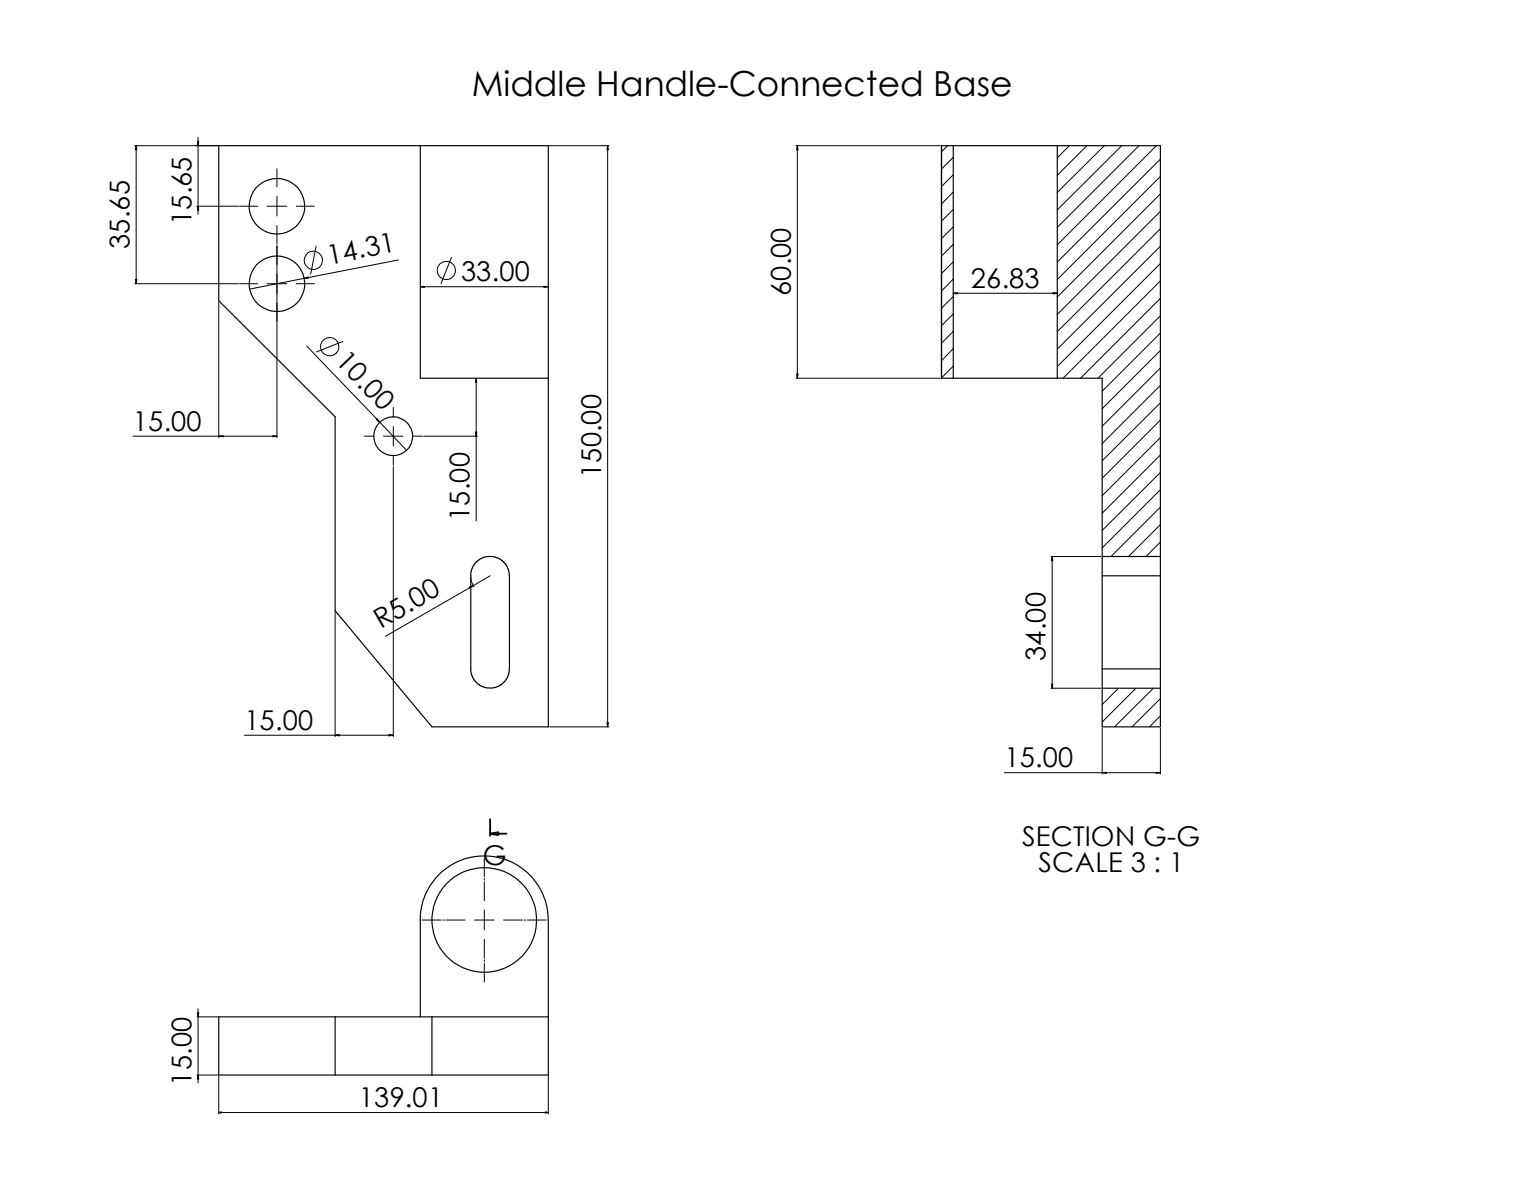
ISO-10303-21;
HEADER;
FILE_DESCRIPTION (('STEP AP214'),
    '1' );
FILE_NAME ('Middle Handle-Connected Base.step',
    '2026-10-26T22:46:44',
    ( '' ),
    ( '' ),
    'SwSTEP 2.0',
    'SolidWorks 2025',
    '' );
FILE_SCHEMA (( 'AUTOMOTIVE_DESIGN' ));
ENDSEC;

DATA;
#80=VECTOR ( 'NONE', #13900, 1000.000000000000227 ) ;
#95=DIRECTION ( 'NONE',  ( -0.5000000000000042188, 0.8660254037844362651, -2.168404344971015524E-16 ) ) ;
#104=EDGE_CURVE ( 'NONE', #402, #10896, #9651, .T. ) ;
#124=CYLINDRICAL_SURFACE ( 'NONE', #4697, 7.155882939242642848 ) ;
#181=EDGE_LOOP ( 'NONE', ( #14178, #14869, #3890, #5041 ) ) ;
#191=ORIENTED_EDGE ( 'NONE', *, *, #11432, .T. ) ;
#206=VERTEX_POINT ( 'NONE', #13865 ) ;
#216=ORIENTED_EDGE ( 'NONE', *, *, #15468, .T. ) ;
#231=DIRECTION ( 'NONE',  ( 0.8660254037844360431, 0.5000000000000044409, -5.976026924694052093E-17 ) ) ;
#281=ORIENTED_EDGE ( 'NONE', *, *, #10002, .F. ) ;
#314=DIRECTION ( 'NONE',  ( 0.5000000000000051070, -0.8660254037844358210, 0.000000000000000000 ) ) ;
#366=ORIENTED_EDGE ( 'NONE', *, *, #15468, .F. ) ;
#398=AXIS2_PLACEMENT_3D ( 'NONE', #14212, #20751, #11112 ) ;
#399=CARTESIAN_POINT ( 'NONE',  ( 77.00490953756757051, 160.5799536996104564, 56.00000000000000711 ) ) ;
#402=VERTEX_POINT ( 'NONE', #14604 ) ;
#403=LINE ( 'NONE', #2101, #20013 ) ;
#458=CARTESIAN_POINT ( 'NONE',  ( 63.15554463217812042, 234.5677573683057062, -19.00000000000000355 ) ) ;
#558=PLANE ( 'NONE',  #15135 ) ;
#564=DIRECTION ( 'NONE',  ( -0.8660254037844359321, -0.5000000000000045519, 5.976026924694053325E-17 ) ) ;
#607=ORIENTED_EDGE ( 'NONE', *, *, #16305, .F. ) ;
#611=CARTESIAN_POINT ( 'NONE',  ( 44.00490953756722945, 217.7376303493834087, -14.00000000000002842 ) ) ;
#722=DIRECTION ( 'NONE',  ( 0.5000000000000042188, -0.8660254037844362651, 1.445602896647343847E-16 ) ) ;
#732=DIRECTION ( 'NONE',  ( 0.000000000000000000, -1.000000000000000000, 2.176694594656153859E-16 ) ) ;
#771=CARTESIAN_POINT ( 'NONE',  ( 22.00490953756706958, 255.8427481158984165, 1.000000000000018208 ) ) ;
#848=ADVANCED_FACE ( 'NONE', ( #20058 ), #558, .F. ) ;
#853=DIRECTION ( 'NONE',  ( -0.5000000000000045519, 0.8660254037844361541, 0.000000000000000000 ) ) ;
#897=ORIENTED_EDGE ( 'NONE', *, *, #5211, .T. ) ;
#898=UNCERTAINTY_MEASURE_WITH_UNIT (LENGTH_MEASURE( 1.000000000000000082E-05 ), #14114, 'distance_accuracy_value', 'NONE');
#903=ORIENTED_EDGE ( 'NONE', *, *, #20153, .T. ) ;
#929=DIRECTION ( 'NONE',  ( -0.8660254037844363761, -0.5000000000000041078, -0.000000000000000000 ) ) ;
#936=CIRCLE ( 'NONE', #18890, 13.50000000000000711 ) ;
#966=EDGE_LOOP ( 'NONE', ( #19200, #16679, #7135, #19433, #20564 ) ) ;
#970=VECTOR ( 'NONE', #19207, 1000.000000000000227 ) ;
#992=EDGE_CURVE ( 'NONE', #997, #5249, #4157, .T. ) ;
#997=VERTEX_POINT ( 'NONE', #771 ) ;
#1026=CARTESIAN_POINT ( 'NONE',  ( 74.05523633728022048, 112.6889375482328717, -12.50000000000000000 ) ) ;
#1127=CIRCLE ( 'NONE', #4512, 7.155882939242646401 ) ;
#1161=ORIENTED_EDGE ( 'NONE', *, *, #19027, .T. ) ;
#1196=EDGE_CURVE ( 'NONE', #9961, #1291, #4537, .T. ) ;
#1200=CYLINDRICAL_SURFACE ( 'NONE', #16859, 5.000000000000033751 ) ;
#1201=VERTEX_POINT ( 'NONE', #3093 ) ;
#1233=FACE_BOUND ( 'NONE', #5689, .T. ) ;
#1259=CARTESIAN_POINT ( 'NONE',  ( 37.00490953756720813, 229.8619860023653132, 26.00000000000001776 ) ) ;
#1274=DIRECTION ( 'NONE',  ( 0.000000000000000000, 0.000000000000000000, 1.000000000000000000 ) ) ;
#1291=VERTEX_POINT ( 'NONE', #4976 ) ;
#1320=EDGE_CURVE ( 'NONE', #8085, #4151, #16435, .T. ) ;
#1358=CARTESIAN_POINT ( 'NONE',  ( 76.19073749086850000, 131.9901410505959518, 41.00000000000001421 ) ) ;
#1365=CARTESIAN_POINT ( 'NONE',  ( 57.00490953756744972, 195.2209698509878990, 11.00000000000001066 ) ) ;
#1416=FACE_BOUND ( 'NONE', #7340, .T. ) ;
#1436=FACE_OUTER_BOUND ( 'NONE', #3782, .T. ) ;
#1538=DIRECTION ( 'NONE',  ( -0.000000000000000000, -0.000000000000000000, 1.000000000000000000 ) ) ;
#1542=CARTESIAN_POINT ( 'NONE',  ( 54.01452848080093361, 170.4004617752990498, 4.000000000000000000 ) ) ;
#1577=ORIENTED_EDGE ( 'NONE', *, *, #12902, .F. ) ;
#1610=CARTESIAN_POINT ( 'NONE',  ( 32.36389338619004263, 157.9004617752989930, -12.50000000000000000 ) ) ;
#1616=EDGE_CURVE ( 'NONE', #1291, #10896, #11018, .T. ) ;
#1617=ORIENTED_EDGE ( 'NONE', *, *, #16795, .T. ) ;
#1641=DIRECTION ( 'NONE',  ( 0.5000000000000044409, -0.8660254037844360431, -0.000000000000000000 ) ) ;
#1651=CARTESIAN_POINT ( 'NONE',  ( 57.02433875312727452, 129.1873174624876413, 41.00000000000001421 ) ) ;
#1654=CARTESIAN_POINT ( 'NONE',  ( 44.05523633727993627, 164.6504617752990498, -12.50000000000000000 ) ) ;
#1656=VERTEX_POINT ( 'NONE', #3646 ) ;
#1676=DIRECTION ( 'NONE',  ( 0.5000000000000051070, -0.8660254037844358210, 0.000000000000000000 ) ) ;
#1741=EDGE_CURVE ( 'NONE', #17881, #8280, #5547, .T. ) ;
#1819=DIRECTION ( 'NONE',  ( 0.8660254037844360431, 0.5000000000000044409, -5.976026924694053325E-17 ) ) ;
#1881=EDGE_CURVE ( 'NONE', #997, #17881, #20600, .T. ) ;
#1891=ORIENTED_EDGE ( 'NONE', *, *, #4582, .T. ) ;
#1918=DIRECTION ( 'NONE',  ( 0.3535533905932770060, -0.6123724356957921389, 0.7071067811865480168 ) ) ;
#1924=VECTOR ( 'NONE', #8304, 1000.000000000000227 ) ;
#1928=CARTESIAN_POINT ( 'NONE',  ( 89.18111854763502322, 139.4901410505960087, 41.00000000000001421 ) ) ;
#1943=( NAMED_UNIT ( * ) SI_UNIT ( $, .STERADIAN. ) SOLID_ANGLE_UNIT ( ) );
#1948=EDGE_CURVE ( 'NONE', #10896, #402, #5560, .T. ) ;
#2017=DIRECTION ( 'NONE',  ( -0.8660254037844359321, -0.5000000000000045519, 5.976026924694053325E-17 ) ) ;
#2094=VECTOR ( 'NONE', #16006, 1000.000000000000227 ) ;
#2101=CARTESIAN_POINT ( 'NONE',  ( 63.15554463217812042, 234.5677573683057062, -8.999999999999973355 ) ) ;
#2108=CARTESIAN_POINT ( 'NONE',  ( 64.01452848080103308, 153.0799536996103996, 56.00000000000000711 ) ) ;
#2201=DIRECTION ( 'NONE',  ( -0.8660254037844361541, -0.5000000000000044409, 5.976026924694052093E-17 ) ) ;
#2204=ORIENTED_EDGE ( 'NONE', *, *, #3642, .F. ) ;
#2214=ORIENTED_EDGE ( 'NONE', *, *, #8610, .T. ) ;
#2232=CYLINDRICAL_SURFACE ( 'NONE', #13515, 13.50000000000000711 ) ;
#2250=VERTEX_POINT ( 'NONE', #7646 ) ;
#2302=DIRECTION ( 'NONE',  ( -0.8660254037844360431, -0.5000000000000045519, -0.000000000000000000 ) ) ;
#2332=CARTESIAN_POINT ( 'NONE',  ( 54.01452848080093361, 170.4004617752990498, 4.000000000000000000 ) ) ;
#2336=CARTESIAN_POINT ( 'NONE',  ( 9.014528480800532151, 248.3427481158983596, -28.99999999999997513 ) ) ;
#2347=DIRECTION ( 'NONE',  ( 0.8660254037844360431, 0.5000000000000044409, -5.976026924694052093E-17 ) ) ;
#2499=ADVANCED_BREP_SHAPE_REPRESENTATION ( '', ( #17599, #18233 ), #10424 ) ;
#2504=EDGE_CURVE ( 'NONE', #10290, #206, #8156, .T. ) ;
#2516=ORIENTED_EDGE ( 'NONE', *, *, #2504, .T. ) ;
#2529=DIRECTION ( 'NONE',  ( 0.8660254037844360431, 0.5000000000000044409, -5.976026924694053325E-17 ) ) ;
#2546=VERTEX_POINT ( 'NONE', #16109 ) ;
#2604=EDGE_LOOP ( 'NONE', ( #4025, #9656 ) ) ;
#2614=DIRECTION ( 'NONE',  ( 0.8660254037844360431, 0.5000000000000044409, -5.976026924694052093E-17 ) ) ;
#2663=FACE_OUTER_BOUND ( 'NONE', #15843, .T. ) ;
#2744=DIRECTION ( 'NONE',  ( 0.5000000000000046629, -0.8660254037844359321, 0.000000000000000000 ) ) ;
#2766=DIRECTION ( 'NONE',  ( 0.5000000000000045519, -0.8660254037844360431, 1.445602896647343354E-16 ) ) ;
#2767=EDGE_CURVE ( 'NONE', #3911, #15566, #15156, .T. ) ;
#2777=ORIENTED_EDGE ( 'NONE', *, *, #7465, .F. ) ;
#2814=DIRECTION ( 'NONE',  ( -0.5000000000000045519, 0.8660254037844361541, 0.000000000000000000 ) ) ;
#2826=ORIENTED_EDGE ( 'NONE', *, *, #9701, .T. ) ;
#2874=ORIENTED_EDGE ( 'NONE', *, *, #12114, .T. ) ;
#2923=CARTESIAN_POINT ( 'NONE',  ( 62.36389338619030553, 105.9389375482328006, -12.50000000000000000 ) ) ;
#2950=DIRECTION ( 'NONE',  ( -1.000000000000000000, 0.000000000000000000, -0.000000000000000000 ) ) ;
#2964=DIRECTION ( 'NONE',  ( 0.5000000000000044409, -0.8660254037844360431, -0.000000000000000000 ) ) ;
#2973=ORIENTED_EDGE ( 'NONE', *, *, #7030, .F. ) ;
#2993=CARTESIAN_POINT ( 'NONE',  ( 60.60228022274862525, 122.9901410505958523, 41.00000000000001421 ) ) ;
#3002=CARTESIAN_POINT ( 'NONE',  ( 127.2868417743716094, 73.48909236273162549, -7.887051853916060842E-15 ) ) ;
#3006=EDGE_LOOP ( 'NONE', ( #12160, #6518, #16180, #7602 ) ) ;
#3053=LINE ( 'NONE', #9507, #2094 ) ;
#3060=AXIS2_PLACEMENT_3D ( 'NONE', #2923, #10751, #12262 ) ;
#3091=VECTOR ( 'NONE', #4986, 1000.000000000000000 ) ;
#3093=CARTESIAN_POINT ( 'NONE',  ( 82.75906001725628869, 150.6134727143929695, 41.00000000000001421 ) ) ;
#3105=FACE_OUTER_BOUND ( 'NONE', #16829, .T. ) ;
#3111=VECTOR ( 'NONE', #18771, 1000.000000000000114 ) ;
#3114=ORIENTED_EDGE ( 'NONE', *, *, #7465, .T. ) ;
#3122=EDGE_CURVE ( 'NONE', #13435, #1201, #10305, .T. ) ;
#3128=CARTESIAN_POINT ( 'NONE',  ( 65.65554463217814885, 230.2376303493835223, -14.00000000000003020 ) ) ;
#3129=CARTESIAN_POINT ( 'NONE',  ( 97.00490953756779788, 125.9389375482329569, 55.99999999999997868 ) ) ;
#3169=( NAMED_UNIT ( * ) SI_UNIT ( $, .STERADIAN. ) SOLID_ANGLE_UNIT ( ) );
#3173=DIRECTION ( 'NONE',  ( 0.8660254037844360431, 0.5000000000000045519, 0.000000000000000000 ) ) ;
#3188=VECTOR ( 'NONE', #2964, 1000.000000000000227 ) ;
#3201=EDGE_CURVE ( 'NONE', #7333, #7908, #12457, .T. ) ;
#3209=EDGE_LOOP ( 'NONE', ( #8623, #12957, #8153, #18833 ) ) ;
#3234=DIRECTION ( 'NONE',  ( -0.8660254037844362651, -0.5000000000000045519, 5.976026924694053325E-17 ) ) ;
#3237=APPLICATION_CONTEXT ( 'automotive_design' ) ;
#3274=DIRECTION ( 'NONE',  ( 0.000000000000000000, -0.000000000000000000, 1.000000000000000000 ) ) ;
#3294=LINE ( 'NONE', #16341, #970 ) ;
#3298=VERTEX_POINT ( 'NONE', #14270 ) ;
#3373=ORIENTED_EDGE ( 'NONE', *, *, #5717, .F. ) ;
#3374=DIRECTION ( 'NONE',  ( -0.8660254037844359321, -0.5000000000000045519, 5.976026924694053325E-17 ) ) ;
#3379=VERTEX_POINT ( 'NONE', #3982 ) ;
#3427=AXIS2_PLACEMENT_3D ( 'NONE', #18271, #12125, #6918 ) ;
#3442=EDGE_CURVE ( 'NONE', #4151, #10290, #12261, .T. ) ;
#3471=CARTESIAN_POINT ( 'NONE',  ( 28.51452848080068847, 214.5677573683055357, -8.999999999999971578 ) ) ;
#3476=EDGE_LOOP ( 'NONE', ( #11530, #16484, #10681, #7077 ) ) ;
#3479=AXIS2_PLACEMENT_3D ( 'NONE', #16291, #8211, #11509 ) ;
#3500=AXIS2_PLACEMENT_3D ( 'NONE', #12737, #7850, #17616 ) ;
#3521=DIRECTION ( 'NONE',  ( 0.000000000000000000, 1.000000000000000000, -1.550730178515671504E-16 ) ) ;
#3555=EDGE_CURVE ( 'NONE', #8280, #12773, #19242, .T. ) ;
#3591=VECTOR ( 'NONE', #6222, 1000.000000000000000 ) ;
#3618=VECTOR ( 'NONE', #8992, 1000.000000000000227 ) ;
#3642=EDGE_CURVE ( 'NONE', #16030, #2546, #10861, .T. ) ;
#3646=CARTESIAN_POINT ( 'NONE',  ( 49.01452848080095492, 179.0607158131434460, 11.00000000000001066 ) ) ;
#3664=CARTESIAN_POINT ( 'NONE',  ( 79.18111854763493795, 156.8106491262847157, 41.00000000000001421 ) ) ;
#3699=ORIENTED_EDGE ( 'NONE', *, *, #8610, .F. ) ;
#3707=CARTESIAN_POINT ( 'NONE',  ( 59.50490953756747103, 190.8908428320656867, 11.00000000000001066 ) ) ;
#3731=CARTESIAN_POINT ( 'NONE',  ( 79.18111854763493795, 156.8106491262847157, 41.00000000000001421 ) ) ;
#3742=VECTOR ( 'NONE', #95, 1000.000000000000114 ) ;
#3743=ORIENTED_EDGE ( 'NONE', *, *, #3442, .F. ) ;
#3753=AXIS2_PLACEMENT_3D ( 'NONE', #6462, #231, #11676 ) ;
#3782=EDGE_LOOP ( 'NONE', ( #6393, #4032, #4528, #3877 ) ) ;
#3851=CARTESIAN_POINT ( 'NONE',  ( 62.00490953756749946, 186.5607158131435028, 11.00000000000001066 ) ) ;
#3877=ORIENTED_EDGE ( 'NONE', *, *, #992, .T. ) ;
#3879=DIRECTION ( 'NONE',  ( -0.5000000000000045519, 0.8660254037844360431, 3.469446951953612710E-16 ) ) ;
#3885=DIRECTION ( 'NONE',  ( 0.8660254037844363761, 0.5000000000000041078, 0.000000000000000000 ) ) ;
#3890=ORIENTED_EDGE ( 'NONE', *, *, #16305, .T. ) ;
#3893=AXIS2_PLACEMENT_3D ( 'NONE', #19737, #564, #5207 ) ;
#3903=ORIENTED_EDGE ( 'NONE', *, *, #2767, .F. ) ;
#3908=AXIS2_PLACEMENT_3D ( 'NONE', #6957, #13552, #18208 ) ;
#3911=VERTEX_POINT ( 'NONE', #9338 ) ;
#3934=EDGE_LOOP ( 'NONE', ( #4702, #19824, #7717, #12186 ) ) ;
#3940=DIRECTION ( 'NONE',  ( 2.052623352751953829E-17, -1.550730178515671504E-16, -1.000000000000000000 ) ) ;
#3957=CIRCLE ( 'NONE', #9361, 5.000000000000008882 ) ;
#3960=ADVANCED_FACE ( 'NONE', ( #12861, #1416, #17739, #9131, #19217 ), #14467, .F. ) ;
#3982=CARTESIAN_POINT ( 'NONE',  ( 54.01452848080093361, 170.4004617752990498, -29.00000000000000000 ) ) ;
#3985=EDGE_LOOP ( 'NONE', ( #13017, #20791, #3373, #8611 ) ) ;
#4025=ORIENTED_EDGE ( 'NONE', *, *, #1948, .T. ) ;
#4032=ORIENTED_EDGE ( 'NONE', *, *, #1741, .F. ) ;
#4048=VECTOR ( 'NONE', #7803, 1000.000000000000227 ) ;
#4049=CARTESIAN_POINT ( 'NONE',  ( 127.2868417743716094, 73.48909236273162549, -8.999999999999934275 ) ) ;
#4059=CARTESIAN_POINT ( 'NONE',  ( 28.51452848080068847, 214.5677573683055357, -19.00000000000000000 ) ) ;
#4103=VECTOR ( 'NONE', #3879, 1000.000000000000227 ) ;
#4151=VERTEX_POINT ( 'NONE', #8483 ) ;
#4157=LINE ( 'NONE', #7641, #4865 ) ;
#4164=ADVANCED_FACE ( 'NONE', ( #12000 ), #13800, .T. ) ;
#4167=DIRECTION ( 'NONE',  ( 0.3535533905932772836, -0.6123724356957930270, -0.7071067811865470176 ) ) ;
#4182=VERTEX_POINT ( 'NONE', #12207 ) ;
#4201=FACE_OUTER_BOUND ( 'NONE', #3006, .T. ) ;
#4288=PRODUCT_DEFINITION_CONTEXT ( 'detailed design', #3237, 'design' ) ;
#4293=ORIENTED_EDGE ( 'NONE', *, *, #4317, .T. ) ;
#4305=DIRECTION ( 'NONE',  ( -0.5000000000000045519, 0.8660254037844361541, 0.000000000000000000 ) ) ;
#4317=EDGE_CURVE ( 'NONE', #2250, #14420, #12495, .T. ) ;
#4351=DIRECTION ( 'NONE',  ( 0.5000000000000051070, -0.8660254037844358210, 0.000000000000000000 ) ) ;
#4430=FACE_OUTER_BOUND ( 'NONE', #14929, .T. ) ;
#4500=VECTOR ( 'NONE', #12225, 1000.000000000000000 ) ;
#4508=EDGE_CURVE ( 'NONE', #1201, #20315, #17654, .T. ) ;
#4512=AXIS2_PLACEMENT_3D ( 'NONE', #7275, #2529, #18847 ) ;
#4528=ORIENTED_EDGE ( 'NONE', *, *, #1881, .F. ) ;
#4537=CIRCLE ( 'NONE', #3500, 13.50000000000000711 ) ;
#4539=DIRECTION ( 'NONE',  ( -0.8660254037844361541, -0.5000000000000044409, 5.976026924694052093E-17 ) ) ;
#4582=EDGE_CURVE ( 'NONE', #4151, #18967, #15361, .T. ) ;
#4617=CARTESIAN_POINT ( 'NONE',  ( 114.2964607176050578, 65.98909236273156864, -7.887051853916060842E-15 ) ) ;
#4650=ORIENTED_EDGE ( 'NONE', *, *, #2504, .F. ) ;
#4671=SHAPE_DEFINITION_REPRESENTATION ( #15533, #6911 ) ;
#4697=AXIS2_PLACEMENT_3D ( 'NONE', #2993, #13057, #20782 ) ;
#4701=CARTESIAN_POINT ( 'NONE',  ( 62.36389338619030553, 105.9389375482328006, -12.50000000000000000 ) ) ;
#4702=ORIENTED_EDGE ( 'NONE', *, *, #15115, .T. ) ;
#4705=VERTEX_POINT ( 'NONE', #17633 ) ;
#4706=CARTESIAN_POINT ( 'NONE',  ( 22.00490953756706958, 255.8427481158984165, 1.000000000000018208 ) ) ;
#4723=EDGE_LOOP ( 'NONE', ( #16715, #12746, #10611, #13018, #5557, #15800 ) ) ;
#4776=AXIS2_PLACEMENT_3D ( 'NONE', #17553, #4305, #6294 ) ;
#4865=VECTOR ( 'NONE', #13704, 1000.000000000000114 ) ;
#4906=( LENGTH_UNIT ( ) NAMED_UNIT ( * ) SI_UNIT ( .MILLI., .METRE. ) );
#4924=EDGE_CURVE ( 'NONE', #9961, #402, #10066, .T. ) ;
#4936=AXIS2_PLACEMENT_3D ( 'NONE', #12174, #9284, #732 ) ;
#4953=EDGE_CURVE ( 'NONE', #1656, #8535, #13488, .T. ) ;
#4956=EDGE_CURVE ( 'NONE', #10290, #19333, #8811, .T. ) ;
#4971=PLANE ( 'NONE',  #14789 ) ;
#4976=CARTESIAN_POINT ( 'NONE',  ( 44.05523633727993627, 164.6504617752990498, -12.50000000000000000 ) ) ;
#4986=DIRECTION ( 'NONE',  ( -0.000000000000000000, -0.000000000000000000, 1.000000000000000000 ) ) ;
#5018=ORIENTED_EDGE ( 'NONE', *, *, #18328, .T. ) ;
#5041=ORIENTED_EDGE ( 'NONE', *, *, #12902, .T. ) ;
#5081=AXIS2_PLACEMENT_3D ( 'NONE', #16688, #8723, #12023 ) ;
#5141=FACE_OUTER_BOUND ( 'NONE', #181, .T. ) ;
#5174=DIRECTION ( 'NONE',  ( -1.000000000000000000, 0.000000000000000000, -0.000000000000000000 ) ) ;
#5207=DIRECTION ( 'NONE',  ( 0.5000000000000051070, -0.8660254037844358210, 0.000000000000000000 ) ) ;
#5211=EDGE_CURVE ( 'NONE', #13758, #20315, #14966, .T. ) ;
#5249=VERTEX_POINT ( 'NONE', #7390 ) ;
#5279=EDGE_LOOP ( 'NONE', ( #13045, #17684, #12503, #2516, #2214, #20077 ) ) ;
#5346=EDGE_LOOP ( 'NONE', ( #4293, #1161, #13965, #19682 ) ) ;
#5388=DIRECTION ( 'NONE',  ( 0.8660254037844362651, 0.5000000000000043299, 0.000000000000000000 ) ) ;
#5398=EDGE_LOOP ( 'NONE', ( #8930, #7080, #9377, #3699, #11160, #7577, #10577, #16346, #8651 ) ) ;
#5408=VECTOR ( 'NONE', #17869, 1000.000000000000000 ) ;
#5457=VERTEX_POINT ( 'NONE', #10786 ) ;
#5543=DIRECTION ( 'NONE',  ( 0.8660254037844361541, 0.5000000000000044409, -5.976026924694052093E-17 ) ) ;
#5547=LINE ( 'NONE', #8531, #20134 ) ;
#5557=ORIENTED_EDGE ( 'NONE', *, *, #15750, .T. ) ;
#5558=ORIENTED_EDGE ( 'NONE', *, *, #11432, .F. ) ;
#5560=CIRCLE ( 'NONE', #13713, 13.50000000000000711 ) ;
#5572=CLOSED_SHELL ( 'NONE', ( #7412, #6367, #18355, #20032, #19598, #9344, #4164, #8946, #7534, #18464, #8305, #12657, #5703, #15409, #20562, #8356, #3960, #9417, #10656, #6638, #6227, #12614, #848, #20649, #14235 ) ) ;
#5573=LINE ( 'NONE', #9176, #7764 ) ;
#5586=EDGE_CURVE ( 'NONE', #17970, #2546, #19309, .T. ) ;
#5620=EDGE_CURVE ( 'NONE', #18365, #3298, #9611, .T. ) ;
#5627=ORIENTED_EDGE ( 'NONE', *, *, #14702, .T. ) ;
#5634=DIRECTION ( 'NONE',  ( -1.632680918566406547E-16, 1.632680918566406547E-16, -1.000000000000000000 ) ) ;
#5689=EDGE_LOOP ( 'NONE', ( #5558, #10487 ) ) ;
#5698=LINE ( 'NONE', #15289, #3618 ) ;
#5703=ADVANCED_FACE ( 'NONE', ( #1436 ), #19036, .F. ) ;
#5717=EDGE_CURVE ( 'NONE', #6944, #997, #11177, .T. ) ;
#5752=AXIS2_PLACEMENT_3D ( 'NONE', #3707, #8160, #10161 ) ;
#5766=PLANE ( 'NONE',  #3060 ) ;
#5774=VECTOR ( 'NONE', #12852, 1000.000000000000114 ) ;
#5819=CARTESIAN_POINT ( 'NONE',  ( 62.00490953756744972, 186.5607158131434744, 26.00000000000001776 ) ) ;
#5821=CARTESIAN_POINT ( 'NONE',  ( 127.2868417743716094, 73.48909236273162549, -18.99999999999997513 ) ) ;
#5826=VECTOR ( 'NONE', #12443, 1000.000000000000114 ) ;
#5842=LINE ( 'NONE', #19006, #4500 ) ;
#5906=CARTESIAN_POINT ( 'NONE',  ( 62.36389338619030553, 105.9389375482328006, -29.00000000000000000 ) ) ;
#5943=LINE ( 'NONE', #15529, #5826 ) ;
#5972=DIRECTION ( 'NONE',  ( 0.000000000000000000, 0.8108848540793840431, -0.5852057359806516201 ) ) ;
#5973=CIRCLE ( 'NONE', #15486, 5.000000000000008882 ) ;
#6154=CARTESIAN_POINT ( 'NONE',  ( 28.51452848080066005, 214.5677573683055357, -8.999999999999969802 ) ) ;
#6165=DIRECTION ( 'NONE',  ( 0.5000000000000026645, -0.8660254037844369313, 0.000000000000000000 ) ) ;
#6222=DIRECTION ( 'NONE',  ( -0.8660254037844363761, -0.5000000000000041078, -0.000000000000000000 ) ) ;
#6223=ORIENTED_EDGE ( 'NONE', *, *, #12130, .T. ) ;
#6227=ADVANCED_FACE ( 'NONE', ( #20888 ), #19312, .F. ) ;
#6238=EDGE_CURVE ( 'NONE', #16821, #5249, #12859, .T. ) ;
#6294=DIRECTION ( 'NONE',  ( -0.8660254037844360431, -0.5000000000000044409, 0.000000000000000000 ) ) ;
#6320=DIRECTION ( 'NONE',  ( 0.5000000000000046629, -0.8660254037844359321, 0.000000000000000000 ) ) ;
#6367=ADVANCED_FACE ( 'NONE', ( #18244 ), #16974, .F. ) ;
#6384=EDGE_CURVE ( 'NONE', #12636, #17110, #10378, .T. ) ;
#6386=DIRECTION ( 'NONE',  ( -0.8660254037844360431, -0.5000000000000046629, 0.000000000000000000 ) ) ;
#6387=ORIENTED_EDGE ( 'NONE', *, *, #11946, .T. ) ;
#6393=ORIENTED_EDGE ( 'NONE', *, *, #12803, .T. ) ;
#6407=FACE_OUTER_BOUND ( 'NONE', #19636, .T. ) ;
#6435=CARTESIAN_POINT ( 'NONE',  ( 22.00490953756706958, 255.8427481158984165, 1.000000000000018208 ) ) ;
#6462=CARTESIAN_POINT ( 'NONE',  ( 30.92607121268107306, 174.3908428320655446, 11.00000000000001243 ) ) ;
#6518=ORIENTED_EDGE ( 'NONE', *, *, #2767, .T. ) ;
#6532=EDGE_LOOP ( 'NONE', ( #11117, #8649, #7240, #11910 ) ) ;
#6542=CARTESIAN_POINT ( 'NONE',  ( 32.36389338619004263, 157.9004617752989930, -29.00000000000000000 ) ) ;
#6546=EDGE_CURVE ( 'NONE', #8080, #4182, #10805, .T. ) ;
#6563=CYLINDRICAL_SURFACE ( 'NONE', #15784, 13.50000000000000711 ) ;
#6622=ORIENTED_EDGE ( 'NONE', *, *, #17520, .F. ) ;
#6638=ADVANCED_FACE ( 'NONE', ( #5141 ), #11731, .F. ) ;
#6653=CARTESIAN_POINT ( 'NONE',  ( 62.00490953756744972, 186.5607158131434744, 26.00000000000001776 ) ) ;
#6808=VECTOR ( 'NONE', #7503, 1000.000000000000114 ) ;
#6864=LINE ( 'NONE', #13349, #20074 ) ;
#6890=DIRECTION ( 'NONE',  ( -0.5000000000000046629, 0.8660254037844359321, 0.000000000000000000 ) ) ;
#6911=SHAPE_REPRESENTATION ( 'Middle Handle-Connected Base', ( #18233 ), #10424 ) ;
#6918=DIRECTION ( 'NONE',  ( 0.5000000000000041078, -0.8660254037844363761, 0.000000000000000000 ) ) ;
#6944=VERTEX_POINT ( 'NONE', #7572 ) ;
#6957=CARTESIAN_POINT ( 'NONE',  ( 62.36389338619030553, 105.9389375482328006, -12.50000000000000000 ) ) ;
#6974=ORIENTED_EDGE ( 'NONE', *, *, #3442, .T. ) ;
#6982=CARTESIAN_POINT ( 'NONE',  ( 41.50490953756720813, 222.0677573683055925, -14.00000000000002842 ) ) ;
#7030=EDGE_CURVE ( 'NONE', #7908, #18515, #12212, .T. ) ;
#7035=( GEOMETRIC_REPRESENTATION_CONTEXT ( 3 ) GLOBAL_UNCERTAINTY_ASSIGNED_CONTEXT ( ( #9765 ) ) GLOBAL_UNIT_ASSIGNED_CONTEXT ( ( #4906, #9671, #1943 ) ) REPRESENTATION_CONTEXT ( 'NONE', 'WORKASPACE' ) );
#7077=ORIENTED_EDGE ( 'NONE', *, *, #1741, .T. ) ;
#7080=ORIENTED_EDGE ( 'NONE', *, *, #8372, .F. ) ;
#7097=CARTESIAN_POINT ( 'NONE',  ( 20.67255043510014900, 151.1504617752989361, -12.49999999999999822 ) ) ;
#7124=EDGE_CURVE ( 'NONE', #11414, #8535, #19633, .T. ) ;
#7135=ORIENTED_EDGE ( 'NONE', *, *, #8504, .F. ) ;
#7159=AXIS2_PLACEMENT_3D ( 'NONE', #13798, #2347, #13373 ) ;
#7161=LINE ( 'NONE', #17134, #4103 ) ;
#7196=ORIENTED_EDGE ( 'NONE', *, *, #8959, .F. ) ;
#7215=CARTESIAN_POINT ( 'NONE',  ( 32.36389338619004263, 157.9004617752989930, -12.50000000000000000 ) ) ;
#7218=CARTESIAN_POINT ( 'NONE',  ( 33.42607121268109438, 170.0607158131433607, 11.00000000000001243 ) ) ;
#7237=LINE ( 'NONE', #20071, #8126 ) ;
#7240=ORIENTED_EDGE ( 'NONE', *, *, #1948, .F. ) ;
#7244=CARTESIAN_POINT ( 'NONE',  ( 64.18022169236998309, 116.7929646387040918, 41.00000000000001421 ) ) ;
#7275=CARTESIAN_POINT ( 'NONE',  ( 89.18111854763502322, 139.4901410505960087, 41.00000000000001421 ) ) ;
#7333=VERTEX_POINT ( 'NONE', #9210 ) ;
#7340=EDGE_LOOP ( 'NONE', ( #10035, #8028 ) ) ;
#7361=EDGE_LOOP ( 'NONE', ( #9059, #5627, #19510, #6223, #216 ) ) ;
#7390=CARTESIAN_POINT ( 'NONE',  ( 9.014528480800532151, 248.3427481158983596, 1.000000000000018208 ) ) ;
#7412=ADVANCED_FACE ( 'NONE', ( #18879 ), #9308, .F. ) ;
#7465=EDGE_CURVE ( 'NONE', #13435, #13758, #11759, .T. ) ;
#7480=VECTOR ( 'NONE', #2302, 1000.000000000000114 ) ;
#7486=AXIS2_PLACEMENT_3D ( 'NONE', #18003, #8120, #1676 ) ;
#7487=EDGE_LOOP ( 'NONE', ( #13412, #8887, #9081, #11780 ) ) ;
#7492=VECTOR ( 'NONE', #16866, 1000.000000000000000 ) ;
#7496=PLANE ( 'NONE',  #4936 ) ;
#7503=DIRECTION ( 'NONE',  ( -0.8660254037844360431, -0.5000000000000045519, -0.000000000000000000 ) ) ;
#7519=CARTESIAN_POINT ( 'NONE',  ( 63.15554463217812042, 234.5677573683057062, -14.00000000000003020 ) ) ;
#7534=ADVANCED_FACE ( 'NONE', ( #8451 ), #16628, .F. ) ;
#7558=EDGE_LOOP ( 'NONE', ( #14179, #13784, #15434, #19801 ) ) ;
#7572=CARTESIAN_POINT ( 'NONE',  ( 22.00490953756706958, 255.8427481158984165, -28.99999999999997513 ) ) ;
#7577=ORIENTED_EDGE ( 'NONE', *, *, #12093, .F. ) ;
#7578=FACE_BOUND ( 'NONE', #966, .T. ) ;
#7580=ORIENTED_EDGE ( 'NONE', *, *, #11443, .F. ) ;
#7602=ORIENTED_EDGE ( 'NONE', *, *, #19091, .T. ) ;
#7641=CARTESIAN_POINT ( 'NONE',  ( 22.00490953756706958, 255.8427481158984165, 1.000000000000018208 ) ) ;
#7646=CARTESIAN_POINT ( 'NONE',  ( 29.50490953756713353, 242.8523670591319785, -19.00000000000000355 ) ) ;
#7700=CARTESIAN_POINT ( 'NONE',  ( 28.42607121268105175, 178.7209698509877285, 11.00000000000001243 ) ) ;
#7711=EDGE_LOOP ( 'NONE', ( #9404, #4650, #3743, #1891 ) ) ;
#7717=ORIENTED_EDGE ( 'NONE', *, *, #4508, .T. ) ;
#7752=LINE ( 'NONE', #17100, #8540 ) ;
#7764=VECTOR ( 'NONE', #722, 1000.000000000000114 ) ;
#7800=VECTOR ( 'NONE', #11342, 1000.000000000000227 ) ;
#7803=DIRECTION ( 'NONE',  ( 0.8660254037844361541, 0.5000000000000044409, -5.976026924694052093E-17 ) ) ;
#7809=CARTESIAN_POINT ( 'NONE',  ( 32.36389338619004263, 157.9004617752989930, 4.000000000000000000 ) ) ;
#7850=DIRECTION ( 'NONE',  ( -0.5000000000000045519, 0.8660254037844361541, 0.000000000000000000 ) ) ;
#7866=DIRECTION ( 'NONE',  ( -0.8660254037844360431, -0.5000000000000045519, 5.976026924694054558E-17 ) ) ;
#7877=EDGE_CURVE ( 'NONE', #4705, #11414, #11001, .T. ) ;
#7888=DIRECTION ( 'NONE',  ( 0.5000000000000045519, -0.8660254037844360431, 0.000000000000000000 ) ) ;
#7908=VERTEX_POINT ( 'NONE', #17775 ) ;
#8028=ORIENTED_EDGE ( 'NONE', *, *, #14866, .F. ) ;
#8052=DIRECTION ( 'NONE',  ( 0.8660254037844362651, 0.5000000000000043299, 0.000000000000000000 ) ) ;
#8080=VERTEX_POINT ( 'NONE', #11732 ) ;
#8085=VERTEX_POINT ( 'NONE', #13533 ) ;
#8110=ORIENTED_EDGE ( 'NONE', *, *, #9143, .T. ) ;
#8120=DIRECTION ( 'NONE',  ( -0.8660254037844362651, -0.5000000000000045519, 5.976026924694053325E-17 ) ) ;
#8126=VECTOR ( 'NONE', #5634, 1000.000000000000000 ) ;
#8132=VECTOR ( 'NONE', #3885, 1000.000000000000000 ) ;
#8153=ORIENTED_EDGE ( 'NONE', *, *, #1616, .T. ) ;
#8156=LINE ( 'NONE', #14668, #5774 ) ;
#8160=DIRECTION ( 'NONE',  ( 0.8660254037844360431, 0.5000000000000044409, -5.976026924694053325E-17 ) ) ;
#8211=DIRECTION ( 'NONE',  ( 0.8660254037844360431, 0.5000000000000044409, -5.976026924694052093E-17 ) ) ;
#8280=VERTEX_POINT ( 'NONE', #15559 ) ;
#8304=DIRECTION ( 'NONE',  ( 0.8660254037844361541, 0.5000000000000044409, -5.976026924694052093E-17 ) ) ;
#8305=ADVANCED_FACE ( 'NONE', ( #20298, #17444 ), #5766, .F. ) ;
#8311=DIRECTION ( 'NONE',  ( -0.8660254037844359321, -0.5000000000000045519, 5.976026924694053325E-17 ) ) ;
#8323=CARTESIAN_POINT ( 'NONE',  ( 16.51452848080062097, 235.3523670591319217, -19.00000000000000355 ) ) ;
#8356=ADVANCED_FACE ( 'NONE', ( #19343 ), #18069, .F. ) ;
#8372=EDGE_CURVE ( 'NONE', #15566, #3379, #16266, .T. ) ;
#8450=CARTESIAN_POINT ( 'NONE',  ( 49.01452848080091229, 179.0607158131434176, 26.00000000000001776 ) ) ;
#8451=FACE_OUTER_BOUND ( 'NONE', #4723, .T. ) ;
#8465=ORIENTED_EDGE ( 'NONE', *, *, #14702, .F. ) ;
#8483=CARTESIAN_POINT ( 'NONE',  ( 77.00490953756757051, 160.5799536996104564, 56.00000000000000711 ) ) ;
#8490=AXIS2_PLACEMENT_3D ( 'NONE', #3664, #10010, #18300 ) ;
#8504=EDGE_CURVE ( 'NONE', #3298, #14420, #15280, .T. ) ;
#8531=CARTESIAN_POINT ( 'NONE',  ( 37.00490953756720813, 229.8619860023653132, 26.00000000000001776 ) ) ;
#8535=VERTEX_POINT ( 'NONE', #3851 ) ;
#8540=VECTOR ( 'NONE', #10722, 1000.000000000000227 ) ;
#8578=DIRECTION ( 'NONE',  ( 0.5000000000000051070, -0.8660254037844358210, 0.000000000000000000 ) ) ;
#8610=EDGE_CURVE ( 'NONE', #206, #17110, #7237, .T. ) ;
#8611=ORIENTED_EDGE ( 'NONE', *, *, #11304, .T. ) ;
#8623=ORIENTED_EDGE ( 'NONE', *, *, #4924, .F. ) ;
#8649=ORIENTED_EDGE ( 'NONE', *, *, #4924, .T. ) ;
#8651=ORIENTED_EDGE ( 'NONE', *, *, #6238, .F. ) ;
#8688=CARTESIAN_POINT ( 'NONE',  ( 32.36389338619004263, 157.9004617752989930, -12.50000000000000000 ) ) ;
#8723=DIRECTION ( 'NONE',  ( -0.8660254037844362651, -0.5000000000000045519, 5.976026924694053325E-17 ) ) ;
#8769=ORIENTED_EDGE ( 'NONE', *, *, #7124, .T. ) ;
#8811=LINE ( 'NONE', #19934, #15923 ) ;
#8843=DIRECTION ( 'NONE',  ( -0.8660254037844360431, -0.5000000000000045519, -0.000000000000000000 ) ) ;
#8887=ORIENTED_EDGE ( 'NONE', *, *, #5620, .T. ) ;
#8930=ORIENTED_EDGE ( 'NONE', *, *, #9256, .F. ) ;
#8946=ADVANCED_FACE ( 'NONE', ( #4430 ), #14205, .F. ) ;
#8959=EDGE_CURVE ( 'NONE', #7333, #14290, #20331, .T. ) ;
#8992=DIRECTION ( 'NONE',  ( 0.5000000000000044409, -0.8660254037844360431, -0.000000000000000000 ) ) ;
#9030=PLANE ( 'NONE',  #10763 ) ;
#9045=ORIENTED_EDGE ( 'NONE', *, *, #12093, .T. ) ;
#9047=DIRECTION ( 'NONE',  ( 0.3841106397986914223, -0.6652991438591137063, 0.6401843996644798196 ) ) ;
#9055=DIRECTION ( 'NONE',  ( -0.5000000000000046629, 0.8660254037844359321, 0.000000000000000000 ) ) ;
#9059=ORIENTED_EDGE ( 'NONE', *, *, #12608, .T. ) ;
#9081=ORIENTED_EDGE ( 'NONE', *, *, #12114, .F. ) ;
#9104=CARTESIAN_POINT ( 'NONE',  ( 62.61279602124705690, 155.5078255381764336, 41.00000000000001421 ) ) ;
#9131=FACE_BOUND ( 'NONE', #19422, .T. ) ;
#9143=EDGE_CURVE ( 'NONE', #19333, #6944, #12915, .T. ) ;
#9164=AXIS2_PLACEMENT_3D ( 'NONE', #20864, #19291, #13326 ) ;
#9176=CARTESIAN_POINT ( 'NONE',  ( 28.51452848080068847, 214.5677573683055357, -19.00000000000000000 ) ) ;
#9208=DIRECTION ( 'NONE',  ( 0.5000000000000051070, -0.8660254037844358210, 0.000000000000000000 ) ) ;
#9210=CARTESIAN_POINT ( 'NONE',  ( 79.76867896048986495, 125.7929646387041771, 41.00000000000001421 ) ) ;
#9256=EDGE_CURVE ( 'NONE', #3379, #16821, #7161, .T. ) ;
#9284=DIRECTION ( 'NONE',  ( -5.666630594370344570E-17, 2.176694594656153859E-16, 1.000000000000000000 ) ) ;
#9308=CYLINDRICAL_SURFACE ( 'NONE', #19206, 5.000000000000008882 ) ;
#9326=CARTESIAN_POINT ( 'NONE',  ( 59.50490953756747103, 190.8908428320656867, 11.00000000000001066 ) ) ;
#9328=AXIS2_PLACEMENT_3D ( 'NONE', #19594, #19398, #314 ) ;
#9338=CARTESIAN_POINT ( 'NONE',  ( 32.36389338619004263, 157.9004617752989930, 4.000000000000000000 ) ) ;
#9344=ADVANCED_FACE ( 'NONE', ( #4201, #10647 ), #15046, .T. ) ;
#9361=AXIS2_PLACEMENT_3D ( 'NONE', #6982, #2017, #8578 ) ;
#9362=CARTESIAN_POINT ( 'NONE',  ( 62.36389338619030553, 105.9389375482328006, -12.50000000000000000 ) ) ;
#9377=ORIENTED_EDGE ( 'NONE', *, *, #11443, .T. ) ;
#9404=ORIENTED_EDGE ( 'NONE', *, *, #11984, .T. ) ;
#9417=ADVANCED_FACE ( 'NONE', ( #7578, #1233, #14070, #14180, #10980 ), #18931, .T. ) ;
#9460=VECTOR ( 'NONE', #11898, 1000.000000000000227 ) ;
#9507=CARTESIAN_POINT ( 'NONE',  ( 54.01452848080093361, 170.4004617752990498, 4.000000000000000000 ) ) ;
#9544=DIRECTION ( 'NONE',  ( 0.8660254037844360431, 0.5000000000000044409, -5.976026924694053325E-17 ) ) ;
#9566=VECTOR ( 'NONE', #2766, 1000.000000000000227 ) ;
#9611=LINE ( 'NONE', #3471, #3742 ) ;
#9619=( NAMED_UNIT ( * ) PLANE_ANGLE_UNIT ( ) SI_UNIT ( $, .RADIAN. ) );
#9651=CIRCLE ( 'NONE', #3908, 13.50000000000000711 ) ;
#9656=ORIENTED_EDGE ( 'NONE', *, *, #104, .T. ) ;
#9671=( NAMED_UNIT ( * ) PLANE_ANGLE_UNIT ( ) SI_UNIT ( $, .RADIAN. ) );
#9700=CARTESIAN_POINT ( 'NONE',  ( 72.61279602124714927, 138.1873174624877265, 41.00000000000001421 ) ) ;
#9701=EDGE_CURVE ( 'NONE', #1656, #4705, #9842, .T. ) ;
#9717=AXIS2_PLACEMENT_3D ( 'NONE', #16812, #2614, #9055 ) ;
#9765=UNCERTAINTY_MEASURE_WITH_UNIT (LENGTH_MEASURE( 1.000000000000000082E-05 ), #4906, 'distance_accuracy_value', 'NONE');
#9829=CARTESIAN_POINT ( 'NONE',  ( 66.19073749086841474, 149.3106491262846589, 41.00000000000001421 ) ) ;
#9839=ORIENTED_EDGE ( 'NONE', *, *, #7877, .F. ) ;
#9842=CIRCLE ( 'NONE', #3427, 5.000000000000005329 ) ;
#9897=CARTESIAN_POINT ( 'NONE',  ( 97.00490953756778367, 125.9389375482329569, -29.00000000000002487 ) ) ;
#9919=ORIENTED_EDGE ( 'NONE', *, *, #6546, .T. ) ;
#9961=VERTEX_POINT ( 'NONE', #7097 ) ;
#9997=CYLINDRICAL_SURFACE ( 'NONE', #3479, 7.155882939242646401 ) ;
#10002=EDGE_CURVE ( 'NONE', #8080, #3911, #13613, .T. ) ;
#10010=DIRECTION ( 'NONE',  ( 0.8660254037844360431, 0.5000000000000044409, -5.976026924694053325E-17 ) ) ;
#10011=EDGE_CURVE ( 'NONE', #8085, #12773, #20240, .T. ) ;
#10035=ORIENTED_EDGE ( 'NONE', *, *, #7124, .F. ) ;
#10066=LINE ( 'NONE', #14884, #20305 ) ;
#10161=DIRECTION ( 'NONE',  ( -0.5000000000000041078, 0.8660254037844363761, 0.000000000000000000 ) ) ;
#10222=ORIENTED_EDGE ( 'NONE', *, *, #4508, .F. ) ;
#10272=ORIENTED_EDGE ( 'NONE', *, *, #4582, .F. ) ;
#10290=VERTEX_POINT ( 'NONE', #13037 ) ;
#10305=LINE ( 'NONE', #15231, #14289 ) ;
#10319=EDGE_LOOP ( 'NONE', ( #191, #16955, #17407, #9839 ) ) ;
#10327=CIRCLE ( 'NONE', #11697, 5.000000000000005329 ) ;
#10371=CARTESIAN_POINT ( 'NONE',  ( 32.36389338619004263, 157.9004617752989930, -12.50000000000000000 ) ) ;
#10378=LINE ( 'NONE', #14987, #7492 ) ;
#10424=( GEOMETRIC_REPRESENTATION_CONTEXT ( 3 ) GLOBAL_UNCERTAINTY_ASSIGNED_CONTEXT ( ( #898 ) ) GLOBAL_UNIT_ASSIGNED_CONTEXT ( ( #14114, #9619, #3169 ) ) REPRESENTATION_CONTEXT ( 'NONE', 'WORKASPACE' ) );
#10463=VECTOR ( 'NONE', #929, 1000.000000000000000 ) ;
#10487=ORIENTED_EDGE ( 'NONE', *, *, #9701, .F. ) ;
#10490=AXIS2_PLACEMENT_3D ( 'NONE', #1928, #1819, #6890 ) ;
#10506=AXIS2_PLACEMENT_3D ( 'NONE', #9829, #3374, #14651 ) ;
#10518=VECTOR ( 'NONE', #1538, 1000.000000000000000 ) ;
#10577=ORIENTED_EDGE ( 'NONE', *, *, #3555, .F. ) ;
#10596=LINE ( 'NONE', #5821, #9566 ) ;
#10611=ORIENTED_EDGE ( 'NONE', *, *, #11304, .F. ) ;
#10647=FACE_BOUND ( 'NONE', #12326, .T. ) ;
#10656=ADVANCED_FACE ( 'NONE', ( #6407 ), #9997, .F. ) ;
#10662=AXIS2_PLACEMENT_3D ( 'NONE', #15710, #8311, #12620 ) ;
#10681=ORIENTED_EDGE ( 'NONE', *, *, #12127, .F. ) ;
#10714=EDGE_CURVE ( 'NONE', #5457, #18365, #403, .T. ) ;
#10722=DIRECTION ( 'NONE',  ( -0.8660254037844361541, -0.5000000000000044409, 5.976026924694052093E-17 ) ) ;
#10751=DIRECTION ( 'NONE',  ( -0.5000000000000045519, 0.8660254037844361541, 0.000000000000000000 ) ) ;
#10763=AXIS2_PLACEMENT_3D ( 'NONE', #12342, #4167, #15532 ) ;
#10786=CARTESIAN_POINT ( 'NONE',  ( 41.50490953756720813, 222.0677573683055925, -8.999999999999971578 ) ) ;
#10805=LINE ( 'NONE', #11129, #80 ) ;
#10820=VECTOR ( 'NONE', #1641, 1000.000000000000114 ) ;
#10853=AXIS2_PLACEMENT_3D ( 'NONE', #7215, #15510, #16976 ) ;
#10855=AXIS2_PLACEMENT_3D ( 'NONE', #1358, #20634, #2744 ) ;
#10861=LINE ( 'NONE', #3128, #13883 ) ;
#10867=VECTOR ( 'NONE', #18706, 1000.000000000000227 ) ;
#10896=VERTEX_POINT ( 'NONE', #1026 ) ;
#10980=FACE_OUTER_BOUND ( 'NONE', #5398, .T. ) ;
#11001=LINE ( 'NONE', #7700, #4048 ) ;
#11018=LINE ( 'NONE', #1654, #3188 ) ;
#11112=DIRECTION ( 'NONE',  ( 0.5000000000000041078, -0.8660254037844363761, 0.000000000000000000 ) ) ;
#11117=ORIENTED_EDGE ( 'NONE', *, *, #17520, .T. ) ;
#11127=DIRECTION ( 'NONE',  ( -0.8660254037844360431, -0.5000000000000044409, 5.976026924694052093E-17 ) ) ;
#11129=CARTESIAN_POINT ( 'NONE',  ( 32.36389338619004263, 157.9004617752989930, -29.00000000000000000 ) ) ;
#11160=ORIENTED_EDGE ( 'NONE', *, *, #11984, .F. ) ;
#11177=LINE ( 'NONE', #4706, #10518 ) ;
#11224=ORIENTED_EDGE ( 'NONE', *, *, #1320, .T. ) ;
#11235=AXIS2_PLACEMENT_3D ( 'NONE', #10371, #853, #20348 ) ;
#11259=DIRECTION ( 'NONE',  ( -0.5000000000000041078, 0.8660254037844363761, 0.000000000000000000 ) ) ;
#11290=DIRECTION ( 'NONE',  ( 0.000000000000000000, 1.000000000000000000, 6.009258394948607529E-16 ) ) ;
#11304=EDGE_CURVE ( 'NONE', #6944, #16821, #20639, .T. ) ;
#11342=DIRECTION ( 'NONE',  ( 0.8660254037844361541, 0.5000000000000044409, -5.976026924694052093E-17 ) ) ;
#11360=CARTESIAN_POINT ( 'NONE',  ( 69.76867896048976547, 143.1134727143928842, 41.00000000000001421 ) ) ;
#11361=CARTESIAN_POINT ( 'NONE',  ( 9.014528480800532151, 248.3427481158983596, 1.000000000000018208 ) ) ;
#11378=CIRCLE ( 'NONE', #9328, 5.000000000000008882 ) ;
#11390=DIRECTION ( 'NONE',  ( -3.469446951953639334E-16, 6.009258394948607529E-16, -1.000000000000000000 ) ) ;
#11414=VERTEX_POINT ( 'NONE', #1365 ) ;
#11415=DIRECTION ( 'NONE',  ( -0.5000000000000045519, 0.8660254037844360431, 3.469446951953612710E-16 ) ) ;
#11417=ORIENTED_EDGE ( 'NONE', *, *, #15115, .F. ) ;
#11432=EDGE_CURVE ( 'NONE', #4705, #1656, #15982, .T. ) ;
#11443=EDGE_CURVE ( 'NONE', #15566, #17110, #3053, .T. ) ;
#11447=DIRECTION ( 'NONE',  ( 0.000000000000000000, 0.000000000000000000, -1.000000000000000000 ) ) ;
#11497=DIRECTION ( 'NONE',  ( 0.5000000000000051070, -0.8660254037844358210, 0.000000000000000000 ) ) ;
#11499=EDGE_CURVE ( 'NONE', #14290, #7333, #16645, .T. ) ;
#11509=DIRECTION ( 'NONE',  ( -0.5000000000000046629, 0.8660254037844359321, 0.000000000000000000 ) ) ;
#11515=ORIENTED_EDGE ( 'NONE', *, *, #12127, .T. ) ;
#11530=ORIENTED_EDGE ( 'NONE', *, *, #3555, .T. ) ;
#11608=EDGE_LOOP ( 'NONE', ( #20354, #2826, #19493, #8769 ) ) ;
#11676=DIRECTION ( 'NONE',  ( -0.5000000000000041078, 0.8660254037844363761, 0.000000000000000000 ) ) ;
#11697=AXIS2_PLACEMENT_3D ( 'NONE', #9326, #9544, #11259 ) ;
#11731=CYLINDRICAL_SURFACE ( 'NONE', #9164, 7.155882939242642848 ) ;
#11732=CARTESIAN_POINT ( 'NONE',  ( 32.36389338619004263, 157.9004617752989930, -29.00000000000000000 ) ) ;
#11759=CIRCLE ( 'NONE', #10506, 7.155882939242646401 ) ;
#11771=CARTESIAN_POINT ( 'NONE',  ( 77.00490953756757051, 160.5799536996104564, 56.00000000000000711 ) ) ;
#11780=ORIENTED_EDGE ( 'NONE', *, *, #12130, .F. ) ;
#11817=PRODUCT_DEFINITION_FORMATION_WITH_SPECIFIED_SOURCE ( 'ANY', '', #17206, .NOT_KNOWN. ) ;
#11898=DIRECTION ( 'NONE',  ( 0.8660254037844361541, 0.5000000000000044409, -5.976026924694052093E-17 ) ) ;
#11910=ORIENTED_EDGE ( 'NONE', *, *, #1616, .F. ) ;
#11946=EDGE_CURVE ( 'NONE', #20315, #1201, #17680, .T. ) ;
#11984=EDGE_CURVE ( 'NONE', #18967, #206, #16571, .T. ) ;
#12000=FACE_OUTER_BOUND ( 'NONE', #14761, .T. ) ;
#12023=DIRECTION ( 'NONE',  ( 0.5000000000000051070, -0.8660254037844358210, 0.000000000000000000 ) ) ;
#12093=EDGE_CURVE ( 'NONE', #12773, #18967, #5842, .T. ) ;
#12114=EDGE_CURVE ( 'NONE', #14274, #3298, #7752, .T. ) ;
#12125=DIRECTION ( 'NONE',  ( -0.8660254037844359321, -0.5000000000000045519, 5.976026924694053325E-17 ) ) ;
#12127=EDGE_CURVE ( 'NONE', #17881, #8085, #5943, .T. ) ;
#12130=EDGE_CURVE ( 'NONE', #5457, #14274, #15421, .T. ) ;
#12160=ORIENTED_EDGE ( 'NONE', *, *, #10002, .T. ) ;
#12174=CARTESIAN_POINT ( 'NONE',  ( 63.15554463217812042, 234.5677573683057062, -8.999999999999973355 ) ) ;
#12183=VECTOR ( 'NONE', #15452, 1000.000000000000000 ) ;
#12186=ORIENTED_EDGE ( 'NONE', *, *, #5211, .F. ) ;
#12207=CARTESIAN_POINT ( 'NONE',  ( 62.36389338619030553, 105.9389375482328006, -29.00000000000000000 ) ) ;
#12212=CIRCLE ( 'NONE', #10490, 7.155882939242646401 ) ;
#12225=DIRECTION ( 'NONE',  ( 0.3535533905932770060, -0.6123724356957921389, 0.7071067811865480168 ) ) ;
#12261=LINE ( 'NONE', #17026, #12183 ) ;
#12262=DIRECTION ( 'NONE',  ( -0.8660254037844360431, -0.5000000000000044409, 0.000000000000000000 ) ) ;
#12326=EDGE_LOOP ( 'NONE', ( #6622, #20757 ) ) ;
#12342=CARTESIAN_POINT ( 'NONE',  ( 77.00490953756757051, 160.5799536996104564, 56.00000000000000711 ) ) ;
#12407=LINE ( 'NONE', #5906, #3591 ) ;
#12443=DIRECTION ( 'NONE',  ( 0.5000000000000044409, -0.8660254037844360431, -0.000000000000000000 ) ) ;
#12453=AXIS2_PLACEMENT_3D ( 'NONE', #9362, #17659, #6386 ) ;
#12455=EDGE_LOOP ( 'NONE', ( #15543, #14516, #18443, #607 ) ) ;
#12457=LINE ( 'NONE', #7244, #10867 ) ;
#12460=CARTESIAN_POINT ( 'NONE',  ( 37.00490953756720813, 229.8619860023653132, 26.00000000000001776 ) ) ;
#12474=ORIENTED_EDGE ( 'NONE', *, *, #8504, .T. ) ;
#12495=LINE ( 'NONE', #15693, #12899 ) ;
#12503=ORIENTED_EDGE ( 'NONE', *, *, #4956, .F. ) ;
#12556=ORIENTED_EDGE ( 'NONE', *, *, #1881, .T. ) ;
#12577=ORIENTED_EDGE ( 'NONE', *, *, #11499, .F. ) ;
#12608=EDGE_CURVE ( 'NONE', #2250, #12799, #10596, .T. ) ;
#12614=ADVANCED_FACE ( 'NONE', ( #2663 ), #20142, .F. ) ;
#12620=DIRECTION ( 'NONE',  ( 0.5000000000000046629, -0.8660254037844359321, 0.000000000000000000 ) ) ;
#12626=CARTESIAN_POINT ( 'NONE',  ( 63.15554463217812042, 234.5677573683057062, -14.00000000000003020 ) ) ;
#12636=VERTEX_POINT ( 'NONE', #13691 ) ;
#12657=ADVANCED_FACE ( 'NONE', ( #19085 ), #16214, .F. ) ;
#12737=CARTESIAN_POINT ( 'NONE',  ( 32.36389338619004263, 157.9004617752989930, -12.50000000000000000 ) ) ;
#12746=ORIENTED_EDGE ( 'NONE', *, *, #9256, .T. ) ;
#12748=DIRECTION ( 'NONE',  ( 0.5000000000000045519, -0.8660254037844361541, -0.000000000000000000 ) ) ;
#12773=VERTEX_POINT ( 'NONE', #8450 ) ;
#12799=VERTEX_POINT ( 'NONE', #14953 ) ;
#12803=EDGE_CURVE ( 'NONE', #5249, #8280, #6864, .T. ) ;
#12852=DIRECTION ( 'NONE',  ( -0.8660254037844360431, -0.5000000000000045519, -0.000000000000000000 ) ) ;
#12859=LINE ( 'NONE', #11361, #3091 ) ;
#12861=FACE_BOUND ( 'NONE', #7361, .T. ) ;
#12899=VECTOR ( 'NONE', #4539, 1000.000000000000227 ) ;
#12902=EDGE_CURVE ( 'NONE', #18515, #7908, #1127, .T. ) ;
#12915=LINE ( 'NONE', #13224, #16616 ) ;
#12957=ORIENTED_EDGE ( 'NONE', *, *, #1196, .T. ) ;
#13017=ORIENTED_EDGE ( 'NONE', *, *, #6238, .T. ) ;
#13018=ORIENTED_EDGE ( 'NONE', *, *, #9143, .F. ) ;
#13037=CARTESIAN_POINT ( 'NONE',  ( 97.00490953756779788, 125.9389375482329569, 55.99999999999997868 ) ) ;
#13045=ORIENTED_EDGE ( 'NONE', *, *, #20153, .F. ) ;
#13057=DIRECTION ( 'NONE',  ( 0.8660254037844360431, 0.5000000000000044409, -5.976026924694052093E-17 ) ) ;
#13065=CIRCLE ( 'NONE', #10662, 7.155882939242646401 ) ;
#13091=CARTESIAN_POINT ( 'NONE',  ( 75.60317707801357301, 163.0078255381764905, 41.00000000000001421 ) ) ;
#13224=CARTESIAN_POINT ( 'NONE',  ( 22.00490953756706958, 255.8427481158984165, -28.99999999999997513 ) ) ;
#13236=CARTESIAN_POINT ( 'NONE',  ( 84.01452848080118940, 118.4389375482329001, 4.000000000000000000 ) ) ;
#13326=DIRECTION ( 'NONE',  ( -0.5000000000000039968, 0.8660254037844363761, 0.000000000000000000 ) ) ;
#13349=CARTESIAN_POINT ( 'NONE',  ( 24.01452848080067071, 222.3619860023652564, 26.00000000000001776 ) ) ;
#13364=ORIENTED_EDGE ( 'NONE', *, *, #1320, .F. ) ;
#13373=DIRECTION ( 'NONE',  ( -0.5000000000000041078, 0.8660254037844363761, 0.000000000000000000 ) ) ;
#13412=ORIENTED_EDGE ( 'NONE', *, *, #10714, .T. ) ;
#13435=VERTEX_POINT ( 'NONE', #11360 ) ;
#13461=CIRCLE ( 'NONE', #12453, 16.50000000000000000 ) ;
#13488=LINE ( 'NONE', #7218, #9460 ) ;
#13504=CARTESIAN_POINT ( 'NONE',  ( 84.01452848080126046, 118.4389375482328859, 55.99999999999997868 ) ) ;
#13515=AXIS2_PLACEMENT_3D ( 'NONE', #8688, #16751, #5388 ) ;
#13527=ORIENTED_EDGE ( 'NONE', *, *, #5586, .T. ) ;
#13533=CARTESIAN_POINT ( 'NONE',  ( 62.00490953756744972, 186.5607158131434744, 26.00000000000001776 ) ) ;
#13552=DIRECTION ( 'NONE',  ( -0.5000000000000045519, 0.8660254037844361541, 0.000000000000000000 ) ) ;
#13566=AXIS2_PLACEMENT_3D ( 'NONE', #3129, #11390, #11290 ) ;
#13584=AXIS2_PLACEMENT_3D ( 'NONE', #7809, #20839, #2950 ) ;
#13613=CIRCLE ( 'NONE', #11235, 16.49999999999999645 ) ;
#13691=CARTESIAN_POINT ( 'NONE',  ( 62.36389338619030553, 105.9389375482328006, 4.000000000000000000 ) ) ;
#13704=DIRECTION ( 'NONE',  ( -0.8660254037844360431, -0.5000000000000045519, -0.000000000000000000 ) ) ;
#13713=AXIS2_PLACEMENT_3D ( 'NONE', #4701, #17648, #14794 ) ;
#13758=VERTEX_POINT ( 'NONE', #9104 ) ;
#13784=ORIENTED_EDGE ( 'NONE', *, *, #3642, .T. ) ;
#13798=CARTESIAN_POINT ( 'NONE',  ( 30.92607121268107306, 174.3908428320655446, 11.00000000000001243 ) ) ;
#13800=CYLINDRICAL_SURFACE ( 'NONE', #10853, 16.49999999999999645 ) ;
#13803=DIRECTION ( 'NONE',  ( 0.5000000000000044409, -0.8660254037844360431, -0.000000000000000000 ) ) ;
#13819=STYLED_ITEM('',(#20967),#17599);
#13865=CARTESIAN_POINT ( 'NONE',  ( 84.01452848080126046, 118.4389375482328859, 55.99999999999997868 ) ) ;
#13883=VECTOR ( 'NONE', #14285, 1000.000000000000227 ) ;
#13900=DIRECTION ( 'NONE',  ( 0.5000000000000044409, -0.8660254037844360431, -0.000000000000000000 ) ) ;
#13965=ORIENTED_EDGE ( 'NONE', *, *, #18328, .F. ) ;
#14020=EDGE_LOOP ( 'NONE', ( #11417, #2777 ) ) ;
#14047=ORIENTED_EDGE ( 'NONE', *, *, #3122, .F. ) ;
#14070=FACE_BOUND ( 'NONE', #16708, .T. ) ;
#14114=( LENGTH_UNIT ( ) NAMED_UNIT ( * ) SI_UNIT ( .MILLI., .METRE. ) );
#14178=ORIENTED_EDGE ( 'NONE', *, *, #3201, .F. ) ;
#14179=ORIENTED_EDGE ( 'NONE', *, *, #16664, .F. ) ;
#14180=FACE_BOUND ( 'NONE', #14020, .T. ) ;
#14205=PLANE ( 'NONE',  #13584 ) ;
#14212=CARTESIAN_POINT ( 'NONE',  ( 46.51452848080092650, 183.3908428320656299, 11.00000000000001066 ) ) ;
#14235=ADVANCED_FACE ( 'NONE', ( #18849 ), #7496, .F. ) ;
#14270=CARTESIAN_POINT ( 'NONE',  ( 16.51452848080062097, 235.3523670591319217, -8.999999999999932498 ) ) ;
#14274=VERTEX_POINT ( 'NONE', #17890 ) ;
#14285=DIRECTION ( 'NONE',  ( -0.8660254037844361541, -0.5000000000000044409, 5.976026924694052093E-17 ) ) ;
#14289=VECTOR ( 'NONE', #5543, 1000.000000000000227 ) ;
#14290=VERTEX_POINT ( 'NONE', #9700 ) ;
#14352=FACE_OUTER_BOUND ( 'NONE', #12455, .T. ) ;
#14420=VERTEX_POINT ( 'NONE', #8323 ) ;
#14467=PLANE ( 'NONE',  #15601 ) ;
#14516=ORIENTED_EDGE ( 'NONE', *, *, #3201, .T. ) ;
#14572=AXIS2_PLACEMENT_3D ( 'NONE', #6542, #3274, #18117 ) ;
#14591=CARTESIAN_POINT ( 'NONE',  ( 49.01452848080091229, 179.0607158131434176, 26.00000000000001776 ) ) ;
#14604=CARTESIAN_POINT ( 'NONE',  ( 50.67255043510042611, 99.18893754823274378, -12.49999999999999822 ) ) ;
#14648=DIRECTION ( 'NONE',  ( 0.5000000000000045519, -0.8660254037844360431, 0.000000000000000000 ) ) ;
#14651=DIRECTION ( 'NONE',  ( 0.5000000000000046629, -0.8660254037844359321, 0.000000000000000000 ) ) ;
#14668=CARTESIAN_POINT ( 'NONE',  ( 97.00490953756779788, 125.9389375482329569, 55.99999999999997868 ) ) ;
#14672=VECTOR ( 'NONE', #18901, 1000.000000000000227 ) ;
#14702=EDGE_CURVE ( 'NONE', #12799, #16030, #15094, .T. ) ;
#14743=VECTOR ( 'NONE', #9047, 1000.000000000000000 ) ;
#14761=EDGE_LOOP ( 'NONE', ( #9919, #903, #18196, #281 ) ) ;
#14789=AXIS2_PLACEMENT_3D ( 'NONE', #6653, #11447, #5174 ) ;
#14794=DIRECTION ( 'NONE',  ( -0.8660254037844362651, -0.5000000000000043299, 0.000000000000000000 ) ) ;
#14811=LINE ( 'NONE', #1651, #1924 ) ;
#14837=CARTESIAN_POINT ( 'NONE',  ( 76.19073749086850000, 131.9901410505959518, 41.00000000000001421 ) ) ;
#14866=EDGE_CURVE ( 'NONE', #8535, #11414, #10327, .T. ) ;
#14869=ORIENTED_EDGE ( 'NONE', *, *, #8959, .T. ) ;
#14870=CARTESIAN_POINT ( 'NONE',  ( 85.60317707801368670, 145.6873174624877834, 41.00000000000001421 ) ) ;
#14884=CARTESIAN_POINT ( 'NONE',  ( 20.67255043510014900, 151.1504617752989361, -12.49999999999999822 ) ) ;
#14929=EDGE_LOOP ( 'NONE', ( #1617, #16897, #7580, #3903 ) ) ;
#14938=DIRECTION ( 'NONE',  ( -0.8660254037844359321, -0.5000000000000045519, 5.976026924694053325E-17 ) ) ;
#14953=CARTESIAN_POINT ( 'NONE',  ( 41.50490953756720813, 222.0677573683055925, -19.00000000000000355 ) ) ;
#14966=LINE ( 'NONE', #19804, #7800 ) ;
#14987=CARTESIAN_POINT ( 'NONE',  ( 62.36389338619030553, 105.9389375482328006, 4.000000000000000000 ) ) ;
#15009=DIRECTION ( 'NONE',  ( 0.5000000000000046629, -0.8660254037844359321, -6.938893903907214573E-16 ) ) ;
#15046=PLANE ( 'NONE',  #4776 ) ;
#15094=CIRCLE ( 'NONE', #3893, 5.000000000000008882 ) ;
#15115=EDGE_CURVE ( 'NONE', #13758, #13435, #13065, .T. ) ;
#15135=AXIS2_PLACEMENT_3D ( 'NONE', #458, #3940, #3521 ) ;
#15156=LINE ( 'NONE', #18415, #8132 ) ;
#15218=FACE_OUTER_BOUND ( 'NONE', #18754, .T. ) ;
#15231=CARTESIAN_POINT ( 'NONE',  ( 54.18022169236989072, 134.1134727143927989, 41.00000000000001421 ) ) ;
#15280=CIRCLE ( 'NONE', #5081, 5.000000000000008882 ) ;
#15289=CARTESIAN_POINT ( 'NONE',  ( 32.36389338619004263, 157.9004617752989930, 4.000000000000000000 ) ) ;
#15322=DIRECTION ( 'NONE',  ( 0.8660254037844360431, 0.5000000000000044409, -5.976026924694053325E-17 ) ) ;
#15323=AXIS2_PLACEMENT_3D ( 'NONE', #14837, #14938, #6320 ) ;
#15361=LINE ( 'NONE', #399, #7480 ) ;
#15409=ADVANCED_FACE ( 'NONE', ( #16431 ), #4971, .F. ) ;
#15421=LINE ( 'NONE', #4049, #14672 ) ;
#15434=ORIENTED_EDGE ( 'NONE', *, *, #16294, .T. ) ;
#15452=DIRECTION ( 'NONE',  ( 0.5000000000000046629, -0.8660254037844359321, -6.938893903907214573E-16 ) ) ;
#15468=EDGE_CURVE ( 'NONE', #14274, #2250, #11378, .T. ) ;
#15473=LINE ( 'NONE', #15573, #10463 ) ;
#15486=AXIS2_PLACEMENT_3D ( 'NONE', #16183, #3234, #11497 ) ;
#15492=ORIENTED_EDGE ( 'NONE', *, *, #4317, .F. ) ;
#15510=DIRECTION ( 'NONE',  ( 0.5000000000000045519, -0.8660254037844361541, -0.000000000000000000 ) ) ;
#15529=CARTESIAN_POINT ( 'NONE',  ( 62.00490953756744972, 186.5607158131434744, 26.00000000000001776 ) ) ;
#15532=DIRECTION ( 'NONE',  ( 0.000000000000000000, 0.7559289460184550613, -0.6546536707079765316 ) ) ;
#15533=PRODUCT_DEFINITION_SHAPE ( 'NONE', 'NONE',  #19104 ) ;
#15543=ORIENTED_EDGE ( 'NONE', *, *, #11499, .T. ) ;
#15559=CARTESIAN_POINT ( 'NONE',  ( 24.01452848080067071, 222.3619860023652564, 26.00000000000001776 ) ) ;
#15566=VERTEX_POINT ( 'NONE', #2332 ) ;
#15573=CARTESIAN_POINT ( 'NONE',  ( 32.36389338619004263, 157.9004617752989930, -29.00000000000000000 ) ) ;
#15601=AXIS2_PLACEMENT_3D ( 'NONE', #3002, #7866, #20793 ) ;
#15693=CARTESIAN_POINT ( 'NONE',  ( 51.15554463217806358, 255.3523670591321206, -19.00000000000000711 ) ) ;
#15710=CARTESIAN_POINT ( 'NONE',  ( 66.19073749086841474, 149.3106491262846589, 41.00000000000001421 ) ) ;
#15750=EDGE_CURVE ( 'NONE', #19333, #4182, #12407, .T. ) ;
#15784=AXIS2_PLACEMENT_3D ( 'NONE', #1610, #12748, #8052 ) ;
#15800=ORIENTED_EDGE ( 'NONE', *, *, #6546, .F. ) ;
#15833=CARTESIAN_POINT ( 'NONE',  ( 51.15554463217806358, 255.3523670591321206, -13.99999999999994671 ) ) ;
#15843=EDGE_LOOP ( 'NONE', ( #2204, #8465, #5018, #13527 ) ) ;
#15903=CARTESIAN_POINT ( 'NONE',  ( 0.000000000000000000, 0.000000000000000000, 0.000000000000000000 ) ) ;
#15923=VECTOR ( 'NONE', #16872, 1000.000000000000000 ) ;
#15940=DIRECTION ( 'NONE',  ( -0.8660254037844360431, -0.5000000000000044409, 5.976026924694052093E-17 ) ) ;
#15982=CIRCLE ( 'NONE', #398, 5.000000000000005329 ) ;
#15983=AXIS2_PLACEMENT_3D ( 'NONE', #4617, #20724, #7888 ) ;
#16006=DIRECTION ( 'NONE',  ( 0.5000000000000044409, -0.8660254037844360431, -0.000000000000000000 ) ) ;
#16030=VERTEX_POINT ( 'NONE', #611 ) ;
#16109=CARTESIAN_POINT ( 'NONE',  ( 31.01452848080070268, 210.2376303493833234, -14.00000000000002842 ) ) ;
#16180=ORIENTED_EDGE ( 'NONE', *, *, #8372, .T. ) ;
#16183=CARTESIAN_POINT ( 'NONE',  ( 28.51452848080068847, 214.5677573683055357, -14.00000000000002842 ) ) ;
#16214=PLANE ( 'NONE',  #19074 ) ;
#16266=LINE ( 'NONE', #1542, #5408 ) ;
#16291=CARTESIAN_POINT ( 'NONE',  ( 50.60228022274853288, 140.3106491262845736, 41.00000000000001421 ) ) ;
#16294=EDGE_CURVE ( 'NONE', #2546, #18365, #5973, .T. ) ;
#16305=EDGE_CURVE ( 'NONE', #14290, #18515, #14811, .T. ) ;
#16333=AXIS2_PLACEMENT_3D ( 'NONE', #3731, #15322, #20066 ) ;
#16341=CARTESIAN_POINT ( 'NONE',  ( 63.15554463217812042, 234.5677573683057062, -19.00000000000000355 ) ) ;
#16346=ORIENTED_EDGE ( 'NONE', *, *, #12803, .F. ) ;
#16431=FACE_OUTER_BOUND ( 'NONE', #3476, .T. ) ;
#16435=LINE ( 'NONE', #11771, #16725 ) ;
#16463=ORIENTED_EDGE ( 'NONE', *, *, #5717, .T. ) ;
#16484=ORIENTED_EDGE ( 'NONE', *, *, #10011, .F. ) ;
#16571=LINE ( 'NONE', #13504, #20712 ) ;
#16616=VECTOR ( 'NONE', #11415, 1000.000000000000227 ) ;
#16628=PLANE ( 'NONE',  #14572 ) ;
#16645=CIRCLE ( 'NONE', #15323, 7.155882939242646401 ) ;
#16664=EDGE_CURVE ( 'NONE', #16030, #5457, #3957, .T. ) ;
#16679=ORIENTED_EDGE ( 'NONE', *, *, #19027, .F. ) ;
#16688=CARTESIAN_POINT ( 'NONE',  ( 16.51452848080062097, 235.3523670591319217, -13.99999999999994493 ) ) ;
#16708=EDGE_LOOP ( 'NONE', ( #12577, #7196 ) ) ;
#16715=ORIENTED_EDGE ( 'NONE', *, *, #19091, .F. ) ;
#16725=VECTOR ( 'NONE', #1918, 1000.000000000000000 ) ;
#16751=DIRECTION ( 'NONE',  ( 0.5000000000000045519, -0.8660254037844361541, -0.000000000000000000 ) ) ;
#16771=APPLICATION_CONTEXT ( 'automotive_design' ) ;
#16795=EDGE_CURVE ( 'NONE', #3911, #12636, #5698, .T. ) ;
#16812=CARTESIAN_POINT ( 'NONE',  ( 50.60228022274853288, 140.3106491262845736, 41.00000000000001421 ) ) ;
#16821=VERTEX_POINT ( 'NONE', #2336 ) ;
#16829=EDGE_LOOP ( 'NONE', ( #2874, #12474, #15492, #366 ) ) ;
#16859=AXIS2_PLACEMENT_3D ( 'NONE', #15833, #15940, #6165 ) ;
#16866=DIRECTION ( 'NONE',  ( 0.8660254037844363761, 0.5000000000000041078, 0.000000000000000000 ) ) ;
#16872=DIRECTION ( 'NONE',  ( -1.632680918566406547E-16, 1.632680918566406547E-16, -1.000000000000000000 ) ) ;
#16897=ORIENTED_EDGE ( 'NONE', *, *, #6384, .T. ) ;
#16955=ORIENTED_EDGE ( 'NONE', *, *, #4953, .T. ) ;
#16974=CYLINDRICAL_SURFACE ( 'NONE', #7159, 5.000000000000005329 ) ;
#16976=DIRECTION ( 'NONE',  ( 0.8660254037844362651, 0.5000000000000038858, 0.000000000000000000 ) ) ;
#17025=AXIS2_PLACEMENT_3D ( 'NONE', #7519, #18876, #9208 ) ;
#17026=CARTESIAN_POINT ( 'NONE',  ( 97.00490953756779788, 125.9389375482329569, 55.99999999999997868 ) ) ;
#17100=CARTESIAN_POINT ( 'NONE',  ( 51.15554463217806358, 255.3523670591321206, -8.999999999999934275 ) ) ;
#17110=VERTEX_POINT ( 'NONE', #13236 ) ;
#17124=CYLINDRICAL_SURFACE ( 'NONE', #9717, 7.155882939242646401 ) ;
#17132=EDGE_LOOP ( 'NONE', ( #8110, #16463, #12556, #11515, #11224, #6974, #20743 ) ) ;
#17134=CARTESIAN_POINT ( 'NONE',  ( 9.014528480800532151, 248.3427481158983596, -28.99999999999997513 ) ) ;
#17206=PRODUCT ( 'Middle Handle-Connected Base', 'Middle Handle-Connected Base', '', ( #17298 ) ) ;
#17237=ORIENTED_EDGE ( 'NONE', *, *, #11946, .F. ) ;
#17298=PRODUCT_CONTEXT ( 'NONE', #16771, 'mechanical' ) ;
#17330=CARTESIAN_POINT ( 'NONE',  ( 32.36389338619004263, 157.9004617752989930, -12.50000000000000000 ) ) ;
#17407=ORIENTED_EDGE ( 'NONE', *, *, #14866, .T. ) ;
#17444=FACE_OUTER_BOUND ( 'NONE', #5279, .T. ) ;
#17520=EDGE_CURVE ( 'NONE', #1291, #9961, #936, .T. ) ;
#17553=CARTESIAN_POINT ( 'NONE',  ( 32.36389338619004263, 157.9004617752989930, -12.50000000000000000 ) ) ;
#17599=MANIFOLD_SOLID_BREP ( 'Cut-Extrude6', #5572 ) ;
#17616=DIRECTION ( 'NONE',  ( -0.8660254037844362651, -0.5000000000000043299, 0.000000000000000000 ) ) ;
#17633=CARTESIAN_POINT ( 'NONE',  ( 44.01452848080091229, 187.7209698509878137, 11.00000000000001066 ) ) ;
#17648=DIRECTION ( 'NONE',  ( -0.5000000000000045519, 0.8660254037844361541, 0.000000000000000000 ) ) ;
#17654=CIRCLE ( 'NONE', #8490, 7.155882939242646401 ) ;
#17659=DIRECTION ( 'NONE',  ( -0.5000000000000045519, 0.8660254037844361541, 0.000000000000000000 ) ) ;
#17680=CIRCLE ( 'NONE', #16333, 7.155882939242646401 ) ;
#17684=ORIENTED_EDGE ( 'NONE', *, *, #15750, .F. ) ;
#17696=EDGE_LOOP ( 'NONE', ( #1577, #2973 ) ) ;
#17702=SHAPE_REPRESENTATION_RELATIONSHIP ( 'NONE' , 'NONE' ,  #6911, #2499 ) ;
#17739=FACE_BOUND ( 'NONE', #17696, .T. ) ;
#17775=CARTESIAN_POINT ( 'NONE',  ( 92.75906001725638816, 133.2929646387042339, 41.00000000000001421 ) ) ;
#17869=DIRECTION ( 'NONE',  ( 0.000000000000000000, 0.000000000000000000, -1.000000000000000000 ) ) ;
#17881=VERTEX_POINT ( 'NONE', #1259 ) ;
#17890=CARTESIAN_POINT ( 'NONE',  ( 29.50490953756714063, 242.8523670591319785, -8.999999999999953815 ) ) ;
#17970=VERTEX_POINT ( 'NONE', #4059 ) ;
#18003=CARTESIAN_POINT ( 'NONE',  ( 28.51452848080068847, 214.5677573683055357, -14.00000000000002842 ) ) ;
#18069=PLANE ( 'NONE',  #13566 ) ;
#18117=DIRECTION ( 'NONE',  ( 1.000000000000000000, 0.000000000000000000, -0.000000000000000000 ) ) ;
#18196=ORIENTED_EDGE ( 'NONE', *, *, #16795, .F. ) ;
#18208=DIRECTION ( 'NONE',  ( -0.8660254037844362651, -0.5000000000000043299, 0.000000000000000000 ) ) ;
#18214=DIRECTION ( 'NONE',  ( 0.3841106397986914223, -0.6652991438591137063, 0.6401843996644798196 ) ) ;
#18233=AXIS2_PLACEMENT_3D ( 'NONE', #15903, #1274, #19656 ) ;
#18244=FACE_OUTER_BOUND ( 'NONE', #10319, .T. ) ;
#18271=CARTESIAN_POINT ( 'NONE',  ( 46.51452848080092650, 183.3908428320656299, 11.00000000000001066 ) ) ;
#18300=DIRECTION ( 'NONE',  ( -0.5000000000000046629, 0.8660254037844359321, 0.000000000000000000 ) ) ;
#18328=EDGE_CURVE ( 'NONE', #12799, #17970, #3294, .T. ) ;
#18355=ADVANCED_FACE ( 'NONE', ( #14352 ), #124, .F. ) ;
#18365=VERTEX_POINT ( 'NONE', #6154 ) ;
#18415=CARTESIAN_POINT ( 'NONE',  ( 32.36389338619004263, 157.9004617752989930, 4.000000000000000000 ) ) ;
#18443=ORIENTED_EDGE ( 'NONE', *, *, #7030, .T. ) ;
#18464=ADVANCED_FACE ( 'NONE', ( #19709 ), #2232, .F. ) ;
#18515=VERTEX_POINT ( 'NONE', #14870 ) ;
#18706=DIRECTION ( 'NONE',  ( 0.8660254037844361541, 0.5000000000000044409, -5.976026924694052093E-17 ) ) ;
#18713=DIRECTION ( 'NONE',  ( -0.8660254037844362651, -0.5000000000000043299, 0.000000000000000000 ) ) ;
#18720=FACE_OUTER_BOUND ( 'NONE', #3934, .T. ) ;
#18754=EDGE_LOOP ( 'NONE', ( #9045, #10272, #13364, #20575 ) ) ;
#18757=CARTESIAN_POINT ( 'NONE',  ( 22.00490953756706958, 255.8427481158984165, -28.99999999999997513 ) ) ;
#18771=DIRECTION ( 'NONE',  ( -0.8660254037844360431, -0.5000000000000045519, -0.000000000000000000 ) ) ;
#18833=ORIENTED_EDGE ( 'NONE', *, *, #104, .F. ) ;
#18847=DIRECTION ( 'NONE',  ( -0.5000000000000046629, 0.8660254037844359321, 0.000000000000000000 ) ) ;
#18849=FACE_OUTER_BOUND ( 'NONE', #7487, .T. ) ;
#18876=DIRECTION ( 'NONE',  ( -0.8660254037844360431, -0.5000000000000044409, 5.976026924694052093E-17 ) ) ;
#18879=FACE_OUTER_BOUND ( 'NONE', #7558, .T. ) ;
#18890=AXIS2_PLACEMENT_3D ( 'NONE', #17330, #2814, #18713 ) ;
#18901=DIRECTION ( 'NONE',  ( -0.5000000000000045519, 0.8660254037844360431, -2.168404344971014538E-16 ) ) ;
#18931=PLANE ( 'NONE',  #15983 ) ;
#18967=VERTEX_POINT ( 'NONE', #2108 ) ;
#19002=AXIS2_PLACEMENT_3D ( 'NONE', #19133, #19240, #5972 ) ;
#19006=CARTESIAN_POINT ( 'NONE',  ( 64.01452848080103308, 153.0799536996103996, 56.00000000000000711 ) ) ;
#19027=EDGE_CURVE ( 'NONE', #14420, #17970, #5573, .T. ) ;
#19036=PLANE ( 'NONE',  #19002 ) ;
#19074=AXIS2_PLACEMENT_3D ( 'NONE', #6435, #14648, #3173 ) ;
#19085=FACE_OUTER_BOUND ( 'NONE', #3985, .T. ) ;
#19091=EDGE_CURVE ( 'NONE', #3379, #8080, #15473, .T. ) ;
#19104=PRODUCT_DEFINITION ( 'UNKNOWN', '', #11817, #4288 ) ;
#19133=CARTESIAN_POINT ( 'NONE',  ( 37.00490953756720813, 229.8619860023653132, 26.00000000000001776 ) ) ;
#19200=ORIENTED_EDGE ( 'NONE', *, *, #5586, .F. ) ;
#19206=AXIS2_PLACEMENT_3D ( 'NONE', #12626, #11127, #4351 ) ;
#19207=DIRECTION ( 'NONE',  ( -0.8660254037844361541, -0.5000000000000044409, 5.976026924694052093E-17 ) ) ;
#19217=FACE_OUTER_BOUND ( 'NONE', #17132, .T. ) ;
#19220=MECHANICAL_DESIGN_GEOMETRIC_PRESENTATION_REPRESENTATION('',(#13819),#7035);
#19240=DIRECTION ( 'NONE',  ( 0.3200921998322428519, -0.5544159532159279591, -0.7682212795973759611 ) ) ;
#19242=LINE ( 'NONE', #14591, #10820 ) ;
#19291=DIRECTION ( 'NONE',  ( 0.8660254037844360431, 0.5000000000000044409, -5.976026924694052093E-17 ) ) ;
#19309=CIRCLE ( 'NONE', #7486, 5.000000000000008882 ) ;
#19312=CYLINDRICAL_SURFACE ( 'NONE', #3753, 5.000000000000005329 ) ;
#19333=VERTEX_POINT ( 'NONE', #9897 ) ;
#19343=FACE_OUTER_BOUND ( 'NONE', #7711, .T. ) ;
#19398=DIRECTION ( 'NONE',  ( -0.8660254037844359321, -0.5000000000000045519, 5.976026924694053325E-17 ) ) ;
#19422=EDGE_LOOP ( 'NONE', ( #17237, #10222 ) ) ;
#19433=ORIENTED_EDGE ( 'NONE', *, *, #5620, .F. ) ;
#19493=ORIENTED_EDGE ( 'NONE', *, *, #7877, .T. ) ;
#19510=ORIENTED_EDGE ( 'NONE', *, *, #16664, .T. ) ;
#19594=CARTESIAN_POINT ( 'NONE',  ( 29.50490953756713353, 242.8523670591319785, -13.99999999999994493 ) ) ;
#19598=ADVANCED_FACE ( 'NONE', ( #20884 ), #6563, .F. ) ;
#19633=CIRCLE ( 'NONE', #5752, 5.000000000000005329 ) ;
#19636=EDGE_LOOP ( 'NONE', ( #14047, #3114, #897, #6387 ) ) ;
#19656=DIRECTION ( 'NONE',  ( 1.000000000000000000, 0.000000000000000000, 0.000000000000000000 ) ) ;
#19682=ORIENTED_EDGE ( 'NONE', *, *, #12608, .F. ) ;
#19709=FACE_OUTER_BOUND ( 'NONE', #3209, .T. ) ;
#19737=CARTESIAN_POINT ( 'NONE',  ( 41.50490953756720813, 222.0677573683055925, -14.00000000000002842 ) ) ;
#19801=ORIENTED_EDGE ( 'NONE', *, *, #10714, .F. ) ;
#19804=CARTESIAN_POINT ( 'NONE',  ( 47.02433875312717504, 146.5078255381763483, 41.00000000000001421 ) ) ;
#19824=ORIENTED_EDGE ( 'NONE', *, *, #3122, .T. ) ;
#19934=CARTESIAN_POINT ( 'NONE',  ( 97.00490953756778367, 125.9389375482329569, -29.00000000000002487 ) ) ;
#20013=VECTOR ( 'NONE', #2201, 1000.000000000000227 ) ;
#20032=ADVANCED_FACE ( 'NONE', ( #18720 ), #17124, .F. ) ;
#20058=FACE_OUTER_BOUND ( 'NONE', #5346, .T. ) ;
#20066=DIRECTION ( 'NONE',  ( -0.5000000000000046629, 0.8660254037844359321, 0.000000000000000000 ) ) ;
#20071=CARTESIAN_POINT ( 'NONE',  ( 84.01452848080124625, 118.4389375482329001, -29.00000000000002487 ) ) ;
#20074=VECTOR ( 'NONE', #18214, 1000.000000000000000 ) ;
#20077=ORIENTED_EDGE ( 'NONE', *, *, #6384, .F. ) ;
#20134=VECTOR ( 'NONE', #8843, 1000.000000000000114 ) ;
#20142=CYLINDRICAL_SURFACE ( 'NONE', #17025, 5.000000000000008882 ) ;
#20153=EDGE_CURVE ( 'NONE', #4182, #12636, #13461, .T. ) ;
#20240=LINE ( 'NONE', #5819, #3111 ) ;
#20298=FACE_BOUND ( 'NONE', #2604, .T. ) ;
#20305=VECTOR ( 'NONE', #13803, 1000.000000000000227 ) ;
#20315=VERTEX_POINT ( 'NONE', #13091 ) ;
#20331=CIRCLE ( 'NONE', #10855, 7.155882939242646401 ) ;
#20348=DIRECTION ( 'NONE',  ( -0.8660254037844362651, -0.5000000000000038858, 0.000000000000000000 ) ) ;
#20354=ORIENTED_EDGE ( 'NONE', *, *, #4953, .F. ) ;
#20562=ADVANCED_FACE ( 'NONE', ( #15218 ), #9030, .F. ) ;
#20564=ORIENTED_EDGE ( 'NONE', *, *, #16294, .F. ) ;
#20575=ORIENTED_EDGE ( 'NONE', *, *, #10011, .T. ) ;
#20600=LINE ( 'NONE', #12460, #14743 ) ;
#20634=DIRECTION ( 'NONE',  ( -0.8660254037844359321, -0.5000000000000045519, 5.976026924694053325E-17 ) ) ;
#20639=LINE ( 'NONE', #18757, #6808 ) ;
#20649=ADVANCED_FACE ( 'NONE', ( #3105 ), #1200, .F. ) ;
#20712=VECTOR ( 'NONE', #15009, 1000.000000000000000 ) ;
#20724=DIRECTION ( 'NONE',  ( -0.8660254037844360431, -0.5000000000000045519, 5.976026924694054558E-17 ) ) ;
#20743=ORIENTED_EDGE ( 'NONE', *, *, #4956, .T. ) ;
#20751=DIRECTION ( 'NONE',  ( -0.8660254037844359321, -0.5000000000000045519, 5.976026924694053325E-17 ) ) ;
#20757=ORIENTED_EDGE ( 'NONE', *, *, #1196, .F. ) ;
#20782=DIRECTION ( 'NONE',  ( -0.5000000000000039968, 0.8660254037844363761, 0.000000000000000000 ) ) ;
#20791=ORIENTED_EDGE ( 'NONE', *, *, #992, .F. ) ;
#20793=DIRECTION ( 'NONE',  ( 0.5000000000000045519, -0.8660254037844360431, 0.000000000000000000 ) ) ;
#20839=DIRECTION ( 'NONE',  ( 0.000000000000000000, 0.000000000000000000, -1.000000000000000000 ) ) ;
#20864=CARTESIAN_POINT ( 'NONE',  ( 60.60228022274862525, 122.9901410505958523, 41.00000000000001421 ) ) ;
#20884=FACE_OUTER_BOUND ( 'NONE', #6532, .T. ) ;
#20888=FACE_OUTER_BOUND ( 'NONE', #11608, .T. ) ;
#20961=COLOUR_RGB('Dark Blue',0.08,0.2,0.34);
#20962=FILL_AREA_STYLE_COLOUR('',#20961);
#20963=FILL_AREA_STYLE('',(#20962));
#20964=SURFACE_STYLE_FILL_AREA(#20963);
#20965=SURFACE_SIDE_STYLE('',(#20964));
#20966=SURFACE_STYLE_USAGE(.BOTH.,#20965);
#20967=PRESENTATION_STYLE_ASSIGNMENT((#20966));
ENDSEC;
END-ISO-10303-21;
